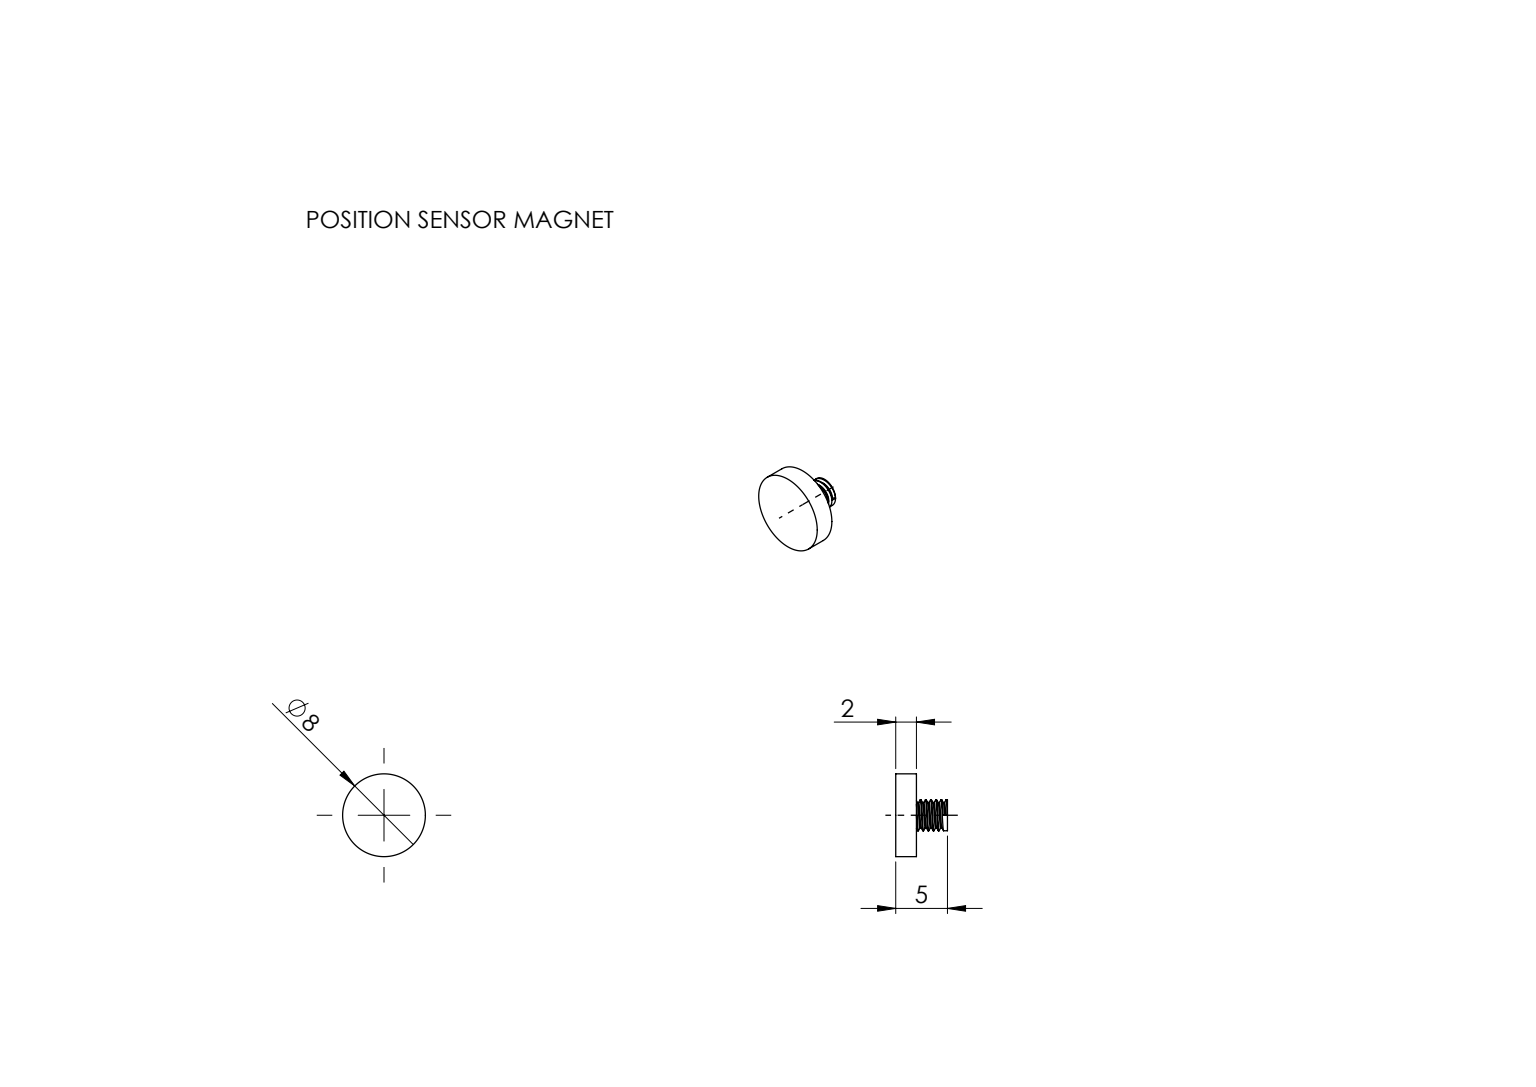
ISO-10303-21;
HEADER;
FILE_DESCRIPTION (('STEP AP214'),
    '1' );
FILE_NAME ('position sensor magnet.step',
    '2026-10-03T18:28:46',
    ( '' ),
    ( '' ),
    'SwSTEP 2.0',
    'SolidWorks 2026',
    '' );
FILE_SCHEMA (( 'AUTOMOTIVE_DESIGN' ));
ENDSEC;

DATA;
#7=EDGE_CURVE ( 'NONE', #9588, #252, #7094, .T. ) ;
#20=CARTESIAN_POINT ( 'NONE',  ( -1.500000000000000222, -13.00000000000000533, -1.812500001365593416 ) ) ;
#22=DIRECTION ( 'NONE',  ( 0.000000000000000000, 0.000000000000000000, 1.000000000000000000 ) ) ;
#32=CARTESIAN_POINT ( 'NONE',  ( -3.181725716174720498E-16, -14.73205080756888385, -1.125000000000000000 ) ) ;
#45=ORIENTED_EDGE ( 'NONE', *, *, #5401, .F. ) ;
#47=CARTESIAN_POINT ( 'NONE',  ( 1.229367062500000163, -13.00000000000000533, 0.2187499993172034862 ) ) ;
#53=CARTESIAN_POINT ( 'NONE',  ( 1.060575238724907038E-16, -11.26794919243112680, 0.06249999863440621611 ) ) ;
#66=CARTESIAN_POINT ( 'NONE',  ( 1.229367062500000385, -12.29022459553277002, -0.8020833340161301894 ) ) ;
#96=( NAMED_UNIT ( * ) PLANE_ANGLE_UNIT ( ) SI_UNIT ( $, .RADIAN. ) );
#98=ORIENTED_EDGE ( 'NONE', *, *, #3375, .T. ) ;
#106=CARTESIAN_POINT ( 'NONE',  ( 1.500000000000000222, -13.00000000000000533, -0.5625000013655934161 ) ) ;
#107=ADVANCED_FACE ( 'NONE', ( #5725 ), #127, .T. ) ;
#113=CARTESIAN_POINT ( 'NONE',  ( 1.060575238724907038E-16, -11.26794919243112680, -0.9375000013655935271 ) ) ;
#116=CARTESIAN_POINT ( 'NONE',  ( 0.6146835312500001924, -11.93533689329915326, -2.760416667349463449 ) ) ;
#127=CYLINDRICAL_SURFACE ( 'NONE', #2700, 1.500000000000000222 ) ;
#135=ORIENTED_EDGE ( 'NONE', *, *, #264, .F. ) ;
#143=CARTESIAN_POINT ( 'NONE',  ( 1.500000000000000222, -13.00000000000000533, 0.000000000000000000 ) ) ;
#148=ADVANCED_FACE ( 'NONE', ( #6475 ), #9031, .T. ) ;
#161=ADVANCED_FACE ( 'NONE', ( #10045 ), #7492, .F. ) ;
#163=CARTESIAN_POINT ( 'NONE',  ( 1.229367062500000163, -13.00000000000000533, -0.3437500006827965970 ) ) ;
#206=CYLINDRICAL_SURFACE ( 'NONE', #9839, 1.500000000000000222 ) ;
#212=CARTESIAN_POINT ( 'NONE',  ( -2.607672531582950546E-16, -14.41955080893447416, -0.3437500006827965415 ) ) ;
#215=EDGE_CURVE ( 'NONE', #8955, #6611, #5198, .T. ) ;
#217=DIRECTION ( 'NONE',  ( 1.000000000000000000, 0.000000000000000000, 0.000000000000000000 ) ) ;
#222=CARTESIAN_POINT ( 'NONE',  ( -1.229367062500000163, -13.70977540446723708, -1.052083334016129967 ) ) ;
#228=DIRECTION ( 'NONE',  ( 1.000000000000000000, 0.000000000000000000, -0.000000000000000000 ) ) ;
#252=VERTEX_POINT ( 'NONE', #2821 ) ;
#260=VECTOR ( 'NONE', #2715, 1000.000000000000000 ) ;
#263=CARTESIAN_POINT ( 'NONE',  ( -2.607672531582950546E-16, -14.41955080893447416, -1.343750000682796708 ) ) ;
#264=EDGE_CURVE ( 'NONE', #5062, #6335, #3411, .T. ) ;
#268=LINE ( 'NONE', #4231, #6080 ) ;
#272=CARTESIAN_POINT ( 'NONE',  ( -1.229367062500000163, -13.00000000000000533, -0.5937500006827968191 ) ) ;
#274=VERTEX_POINT ( 'NONE', #5981 ) ;
#276=DIRECTION ( 'NONE',  ( 1.000000000000000000, 0.000000000000000000, 0.000000000000000000 ) ) ;
#279=CARTESIAN_POINT ( 'NONE',  ( 0.9270509719278221539, -11.80318232062615991, 0.01099716686063855267 ) ) ;
#289=CARTESIAN_POINT ( 'NONE',  ( -1.229367062500000163, -13.00000000000000533, -1.468750000682796486 ) ) ;
#301=CARTESIAN_POINT ( 'NONE',  ( -1.229367062500000163, -13.00000000000000533, -2.593750000682796486 ) ) ;
#312=CARTESIAN_POINT ( 'NONE',  ( 8.692241771943169307E-17, -11.58044919106553294, -0.09375000068279677745 ) ) ;
#320=CARTESIAN_POINT ( 'NONE',  ( -2.607672531582950546E-16, -14.41955080893447416, -0.4687500006827967081 ) ) ;
#334=CARTESIAN_POINT ( 'NONE',  ( 1.229367062499999719, -13.70977540446724063, -2.260416667349463005 ) ) ;
#336=CARTESIAN_POINT ( 'NONE',  ( -2.607672531582950546E-16, -14.41955080893447416, -0.3437500006827965415 ) ) ;
#339=ORIENTED_EDGE ( 'NONE', *, *, #9880, .F. ) ;
#343=EDGE_CURVE ( 'NONE', #9521, #8355, #5353, .T. ) ;
#351=CARTESIAN_POINT ( 'NONE',  ( -0.6146835312500006365, -14.06466310670085562, -0.01041666734946352160 ) ) ;
#366=CARTESIAN_POINT ( 'NONE',  ( 1.229367062500000163, -13.00000000000000533, -2.218750000682796486 ) ) ;
#367=EDGE_LOOP ( 'NONE', ( #135, #7776, #8041, #9114 ) ) ;
#374=CARTESIAN_POINT ( 'NONE',  ( -1.229367062500000163, -12.29022459553277002, -2.635416667349463449 ) ) ;
#389=CARTESIAN_POINT ( 'NONE',  ( 1.229367062500000163, -13.00000000000000533, -1.718750000682796486 ) ) ;
#401=CARTESIAN_POINT ( 'NONE',  ( 1.229367062500000163, -13.00000000000000533, 0.1562499993172034307 ) ) ;
#415=( BOUNDED_CURVE ( )  B_SPLINE_CURVE ( 2, ( #2838, #7109, #4670, #2788, #2741, #9258, #6005 ),
 .UNSPECIFIED., .F., .T. ) 
 B_SPLINE_CURVE_WITH_KNOTS ( ( 3, 2, 2, 3 ),
 ( 0.7500000000000000000, 0.7777777777777777901, 0.8055555555555554692, 0.8333333333333332593 ),
 .UNSPECIFIED. ) 
 CURVE ( )  GEOMETRIC_REPRESENTATION_ITEM ( )  RATIONAL_B_SPLINE_CURVE ( ( 1.000000000000000000, 0.8660254037844387076, 1.000000000000000000, 0.8660254037844387076, 1.000000000000000000, 0.8660254037844392627, 0.9999999999999994449 ) ) 
 REPRESENTATION_ITEM ( '' )  );
#416=CARTESIAN_POINT ( 'NONE',  ( -1.500000000000000222, -13.00000000000000533, -1.312500001365593416 ) ) ;
#428=AXIS2_PLACEMENT_3D ( 'NONE', #1380, #3660, #8440 ) ;
#439=CARTESIAN_POINT ( 'NONE',  ( 1.229367062500000385, -12.29022459553277002, -1.677083334016129967 ) ) ;
#452=CARTESIAN_POINT ( 'NONE',  ( 0.7500000000000003331, -11.70096189432334732, -2.916666666666666963 ) ) ;
#487=CARTESIAN_POINT ( 'NONE',  ( -2.607672531582950546E-16, -14.41955080893447416, -1.968750000682796708 ) ) ;
#489=CARTESIAN_POINT ( 'NONE',  ( 8.692241771943170539E-17, -11.58044919106553650, -1.593750000682796708 ) ) ;
#499=CARTESIAN_POINT ( 'NONE',  ( -1.229367062500000385, -13.70977540446723886, -1.552083334016130189 ) ) ;
#517=CARTESIAN_POINT ( 'NONE',  ( 1.499999999999999778, -13.86602540378444637, -2.541666666666666963 ) ) ;
#531=CARTESIAN_POINT ( 'NONE',  ( 1.229367062500000163, -13.00000000000000533, -2.718750000682796486 ) ) ;
#534=CARTESIAN_POINT ( 'NONE',  ( -1.500000000000000666, -13.86602540378444637, -0.2083333333333333703 ) ) ;
#540=CARTESIAN_POINT ( 'NONE',  ( 1.229367062500000385, -12.29022459553277002, -1.802083334016129967 ) ) ;
#543=CARTESIAN_POINT ( 'NONE',  ( -1.229367062500000163, -12.29022459553277002, -1.010416667349463227 ) ) ;
#554=CARTESIAN_POINT ( 'NONE',  ( -0.6146835312500006365, -14.06466310670085562, -1.010416667349463227 ) ) ;
#560=ORIENTED_EDGE ( 'NONE', *, *, #5898, .F. ) ;
#564=CARTESIAN_POINT ( 'NONE',  ( 1.500000000000000222, -12.13397459621556784, -1.458333333333333481 ) ) ;
#581=( GEOMETRIC_REPRESENTATION_CONTEXT ( 3 ) GLOBAL_UNCERTAINTY_ASSIGNED_CONTEXT ( ( #4844 ) ) GLOBAL_UNIT_ASSIGNED_CONTEXT ( ( #7026, #8784, #10332 ) ) REPRESENTATION_CONTEXT ( 'NONE', 'WORKASPACE' ) );
#588=CARTESIAN_POINT ( 'NONE',  ( -2.607672531582950546E-16, -14.41955080893447416, -2.468750000682796486 ) ) ;
#606=CARTESIAN_POINT ( 'NONE',  ( -0.7500000000000007772, -14.29903810567666156, -1.666666666666666741 ) ) ;
#639=CARTESIAN_POINT ( 'NONE',  ( -1.229367062500000163, -13.00000000000000533, 0.03124999931720332663 ) ) ;
#647=CARTESIAN_POINT ( 'NONE',  ( 1.500000000000000222, -13.00000000000000533, 0.4374999986344065284 ) ) ;
#650=ORIENTED_EDGE ( 'NONE', *, *, #2389, .T. ) ;
#655=CARTESIAN_POINT ( 'NONE',  ( 1.500000000000000222, -13.00000000000000533, -1.500000000000000000 ) ) ;
#665=CARTESIAN_POINT ( 'NONE',  ( 0.000000000000000000, -13.00000000000000533, -3.000000000000000000 ) ) ;
#679=ORIENTED_EDGE ( 'NONE', *, *, #5695, .T. ) ;
#685=CARTESIAN_POINT ( 'NONE',  ( 0.7500000000000003331, -11.70096189432334732, 0.02083333196773980503 ) ) ;
#687=CARTESIAN_POINT ( 'NONE',  ( -1.500000000000000222, -13.00000000000000533, -0.3125000013655936937 ) ) ;
#690=ORIENTED_EDGE ( 'NONE', *, *, #6660, .T. ) ;
#700=CARTESIAN_POINT ( 'NONE',  ( 0.6146835312499993043, -14.06466310670085562, 0.1979166659838698661 ) ) ;
#708=EDGE_LOOP ( 'NONE', ( #5948, #2687, #4855, #10434, #9641, #7515, #7392, #3265, #7780, #4226, #690, #4016, #8469, #9796, #6235 ) ) ;
#716=CARTESIAN_POINT ( 'NONE',  ( 0.7500000000000003331, -11.70096189432334732, -0.9166666666666667407 ) ) ;
#740=CARTESIAN_POINT ( 'NONE',  ( -0.7499999999999997780, -11.70096189432334555, -0.3958333346989269530 ) ) ;
#741=CIRCLE ( 'NONE', #9725, 4.000000000000000000 ) ;
#748=EDGE_CURVE ( 'NONE', #10270, #6751, #4270, .T. ) ;
#758=DIRECTION ( 'NONE',  ( 0.000000000000000000, 0.000000000000000000, 1.000000000000000000 ) ) ;
#764=DIRECTION ( 'NONE',  ( 1.000000000000000000, 0.000000000000000000, 0.000000000000000000 ) ) ;
#768=CARTESIAN_POINT ( 'NONE',  ( 1.060575238724907038E-16, -11.26794919243112680, -0.8750000000000004441 ) ) ;
#774=CIRCLE ( 'NONE', #8227, 1.500000000000000222 ) ;
#775=CARTESIAN_POINT ( 'NONE',  ( 1.500000000000000222, -12.13397459621556784, -2.520833334698926897 ) ) ;
#788=CARTESIAN_POINT ( 'NONE',  ( -1.499999999999998224, -12.13397459621556607, -1.791666666666667185 ) ) ;
#794=CARTESIAN_POINT ( 'NONE',  ( 1.500000000000000444, -12.13397459621556607, -0.5208333346989270085 ) ) ;
#797=ADVANCED_FACE ( 'NONE', ( #10440 ), #5240, .T. ) ;
#806=CARTESIAN_POINT ( 'NONE',  ( -0.6146835312499998594, -11.93533689329915326, -0.6770833340161300784 ) ) ;
#815=CARTESIAN_POINT ( 'NONE',  ( 0.000000000000000000, -13.00000000000000533, 0.000000000000000000 ) ) ;
#819=CARTESIAN_POINT ( 'NONE',  ( -1.500000000000000000, -12.13397459621556607, -1.791666666666666741 ) ) ;
#820=ORIENTED_EDGE ( 'NONE', *, *, #940, .F. ) ;
#828=EDGE_CURVE ( 'NONE', #5863, #2098, #3844, .T. ) ;
#829=VECTOR ( 'NONE', #7182, 1000.000000000000227 ) ;
#844=CARTESIAN_POINT ( 'NONE',  ( -1.500000000000000666, -13.86602540378444459, -0.2708333346989268420 ) ) ;
#849=CARTESIAN_POINT ( 'NONE',  ( -1.500000000000000222, -13.00000000000000533, -0.8125000013655935271 ) ) ;
#859=EDGE_CURVE ( 'NONE', #6218, #8785, #9534, .T. ) ;
#860=CARTESIAN_POINT ( 'NONE',  ( -2.607672531582950546E-16, -14.41955080893447416, -0.9687500006827967081 ) ) ;
#871=AXIS2_PLACEMENT_3D ( 'NONE', #3735, #4797, #7928 ) ;
#879=CARTESIAN_POINT ( 'NONE',  ( -0.6146835312499998594, -11.93533689329915326, -2.552083334016129967 ) ) ;
#884=ORIENTED_EDGE ( 'NONE', *, *, #6432, .T. ) ;
#885=EDGE_CURVE ( 'NONE', #4827, #274, #3898, .T. ) ;
#898=CARTESIAN_POINT ( 'NONE',  ( -1.500000000000000222, -13.00000000000000533, -1.312500001365593416 ) ) ;
#904=FACE_OUTER_BOUND ( 'NONE', #4621, .T. ) ;
#907=CARTESIAN_POINT ( 'NONE',  ( 1.229367062500000163, -12.29022459553277002, -2.802083334016129967 ) ) ;
#910=CARTESIAN_POINT ( 'NONE',  ( -1.229367062500000163, -12.29022459553277002, -1.135416667349463227 ) ) ;
#927=( GEOMETRIC_REPRESENTATION_CONTEXT ( 3 ) GLOBAL_UNCERTAINTY_ASSIGNED_CONTEXT ( ( #6427 ) ) GLOBAL_UNIT_ASSIGNED_CONTEXT ( ( #1683, #96, #6600 ) ) REPRESENTATION_CONTEXT ( 'NONE', 'WORKASPACE' ) );
#938=CARTESIAN_POINT ( 'NONE',  ( 1.499999999999999778, -13.86602540378444637, -1.104166668032260379 ) ) ;
#940=EDGE_CURVE ( 'NONE', #2098, #9635, #9900, .T. ) ;
#958=ORIENTED_EDGE ( 'NONE', *, *, #5876, .F. ) ;
#960=CARTESIAN_POINT ( 'NONE',  ( 0.6146835312499993043, -14.06466310670085562, -1.427083334016129967 ) ) ;
#987=CARTESIAN_POINT ( 'NONE',  ( 1.500000000000000222, -13.00000000000000533, -1.062500001365593416 ) ) ;
#988=ORIENTED_EDGE ( 'NONE', *, *, #5006, .F. ) ;
#989=ORIENTED_EDGE ( 'NONE', *, *, #6351, .F. ) ;
#997=CARTESIAN_POINT ( 'NONE',  ( -0.6146835312499998594, -11.93533689329915326, -0.5520833340161299674 ) ) ;
#1006=CARTESIAN_POINT ( 'NONE',  ( 1.229367062500000163, -13.00000000000000533, -0.8437500006827965970 ) ) ;
#1017=FACE_OUTER_BOUND ( 'NONE', #1736, .T. ) ;
#1020=CARTESIAN_POINT ( 'NONE',  ( -1.229367062500000163, -12.29022459553277002, -1.510416667349463227 ) ) ;
#1030=AXIS2_PLACEMENT_3D ( 'NONE', #8223, #1546, #7416 ) ;
#1033=EDGE_CURVE ( 'NONE', #1639, #6225, #3260, .T. ) ;
#1042=CARTESIAN_POINT ( 'NONE',  ( 1.229367062500000163, -13.00000000000000533, -2.343750000682796486 ) ) ;
#1054=CARTESIAN_POINT ( 'NONE',  ( -1.229367062500000163, -13.00000000000000533, -1.468750000682796486 ) ) ;
#1061=VERTEX_POINT ( 'NONE', #6314 ) ;
#1063=CARTESIAN_POINT ( 'NONE',  ( -1.229367062500000163, -12.29022459553277002, -0.6354166673494632267 ) ) ;
#1074=CARTESIAN_POINT ( 'NONE',  ( 1.500000000000000222, -13.00000000000000533, -3.000000000000000000 ) ) ;
#1076=CARTESIAN_POINT ( 'NONE',  ( 0.6146835312500001924, -11.93533689329915326, -2.135416667349463449 ) ) ;
#1079=CARTESIAN_POINT ( 'NONE',  ( 1.229367062500000163, -13.00000000000000533, -2.218750000682796486 ) ) ;
#1089=CARTESIAN_POINT ( 'NONE',  ( 1.229367062500000385, -12.29022459553277002, -2.802083334016129523 ) ) ;
#1095=CARTESIAN_POINT ( 'NONE',  ( -1.500000000000000222, -13.00000000000000533, -0.2500000000000002220 ) ) ;
#1101=CARTESIAN_POINT ( 'NONE',  ( 8.692241771943169307E-17, -11.58044919106553294, -1.593750000682796486 ) ) ;
#1106=CARTESIAN_POINT ( 'NONE',  ( -1.500000000000000222, -13.00000000000000533, -2.750000000000000000 ) ) ;
#1107=CARTESIAN_POINT ( 'NONE',  ( -1.499999999999996669, -12.13397459621556607, -0.8541666680322607119 ) ) ;
#1112=CARTESIAN_POINT ( 'NONE',  ( -1.229367062500000163, -13.00000000000000533, -2.093750000682796930 ) ) ;
#1128=CARTESIAN_POINT ( 'NONE',  ( 0.6146835312500001924, -11.93533689329915326, -1.135416667349463227 ) ) ;
#1131=CARTESIAN_POINT ( 'NONE',  ( 0.6146835312499993043, -14.06466310670085562, -1.802083334016129745 ) ) ;
#1151=CARTESIAN_POINT ( 'NONE',  ( -2.607672531582950546E-16, -14.41955080893447416, 0.1562499993172034585 ) ) ;
#1152=EDGE_CURVE ( 'NONE', #4358, #7070, #4378, .T. ) ;
#1160=CARTESIAN_POINT ( 'NONE',  ( -1.229367062500000163, -13.00000000000000533, -1.593750000682796708 ) ) ;
#1176=CARTESIAN_POINT ( 'NONE',  ( -0.6146835312500006365, -14.06466310670085562, -0.8854166673494632267 ) ) ;
#1178=CARTESIAN_POINT ( 'NONE',  ( -1.229367062500000163, -13.00000000000000533, -0.4687500006827967081 ) ) ;
#1181=COLOUR_RGB ( '', 0.09019608, 0.27058824, 0.51372549) ;
#1192=CARTESIAN_POINT ( 'NONE',  ( 0.6146835312499993043, -14.06466310670085562, 0.07291666598386974119 ) ) ;
#1195=VECTOR ( 'NONE', #7864, 1000.000000000000000 ) ;
#1202=ORIENTED_EDGE ( 'NONE', *, *, #1450, .T. ) ;
#1229=CARTESIAN_POINT ( 'NONE',  ( -0.6146835312499998594, -11.93533689329915326, -2.052083334016129967 ) ) ;
#1231=CARTESIAN_POINT ( 'NONE',  ( -0.6146835312499998594, -11.93533689329915326, -2.052083334016129967 ) ) ;
#1246=CARTESIAN_POINT ( 'NONE',  ( -0.6146835312499998594, -11.93533689329915326, -0.1770833340161300506 ) ) ;
#1261=ORIENTED_EDGE ( 'NONE', *, *, #9693, .T. ) ;
#1264=DIRECTION ( 'NONE',  ( 1.000000000000000000, 0.000000000000000000, 0.000000000000000000 ) ) ;
#1276=PRODUCT_DEFINITION ( 'UNKNOWN', '', #9579, #7173 ) ;
#1282=CARTESIAN_POINT ( 'NONE',  ( -1.229367062500000163, -12.29022459553277002, -0.01041666734946308792 ) ) ;
#1284=CARTESIAN_POINT ( 'NONE',  ( 1.229367062500000163, -13.00000000000000533, -0.2187500006827964583 ) ) ;
#1294=PRESENTATION_STYLE_ASSIGNMENT (( #8606 ) ) ;
#1296=CARTESIAN_POINT ( 'NONE',  ( -0.6146835312500006365, -14.06466310670085562, -2.010416667349463005 ) ) ;
#1312=DIRECTION ( 'NONE',  ( 0.000000000000000000, 0.000000000000000000, 1.000000000000000000 ) ) ;
#1328=CARTESIAN_POINT ( 'NONE',  ( -0.6146835312500006365, -14.06466310670085562, 0.1145833326505365929 ) ) ;
#1330=CARTESIAN_POINT ( 'NONE',  ( -1.229367062500000163, -13.70977540446723708, -1.427083334016129745 ) ) ;
#1341=ADVANCED_FACE ( 'NONE', ( #6840 ), #10110, .T. ) ;
#1346=CARTESIAN_POINT ( 'NONE',  ( 1.229367062500000385, -12.29022459553277002, -1.302083334016129967 ) ) ;
#1365=DIRECTION ( 'NONE',  ( 0.000000000000000000, 0.000000000000000000, 1.000000000000000000 ) ) ;
#1366=AXIS2_PLACEMENT_3D ( 'NONE', #3051, #8669, #1515 ) ;
#1372=VERTEX_POINT ( 'NONE', #8916 ) ;
#1380=CARTESIAN_POINT ( 'NONE',  ( 0.000000000000000000, -13.00000000000000533, -3.000000000000000000 ) ) ;
#1386=CARTESIAN_POINT ( 'NONE',  ( 0.6146835312499993043, -14.06466310670085562, -1.927083334016129967 ) ) ;
#1400=CARTESIAN_POINT ( 'NONE',  ( 1.500000000000000000, -13.86602540378444459, -0.04166666666666684476 ) ) ;
#1424=CARTESIAN_POINT ( 'NONE',  ( 1.060575238724907038E-16, -11.26794919243112680, -1.937500001365593416 ) ) ;
#1427=( BOUNDED_CURVE ( )  B_SPLINE_CURVE ( 2, ( #7646, #9285, #7539, #8545, #9987, #1871, #8394 ),
 .UNSPECIFIED., .F., .T. ) 
 B_SPLINE_CURVE_WITH_KNOTS ( ( 3, 2, 2, 3 ),
 ( 0.1666666666666666574, 0.1944444444444444475, 0.2222222222222222099, 0.2500000000000000000 ),
 .UNSPECIFIED. ) 
 CURVE ( )  GEOMETRIC_REPRESENTATION_ITEM ( )  RATIONAL_B_SPLINE_CURVE ( ( 1.000000000000000000, 0.8660254037844387076, 1.000000000000000000, 0.8660254037844387076, 1.000000000000000000, 0.8660254037844387076, 1.000000000000000000 ) ) 
 REPRESENTATION_ITEM ( '' )  );
#1433=VECTOR ( 'NONE', #6619, 1000.000000000000000 ) ;
#1438=CARTESIAN_POINT ( 'NONE',  ( 1.229367062500000385, -12.29022459553277002, -0.6770833340161300784 ) ) ;
#1450=EDGE_CURVE ( 'NONE', #7070, #4358, #9157, .T. ) ;
#1453=AXIS2_PLACEMENT_3D ( 'NONE', #4245, #22, #5722 ) ;
#1456=CARTESIAN_POINT ( 'NONE',  ( -0.7499999999999997780, -11.70096189432334555, -0.8333333333333334814 ) ) ;
#1465=CARTESIAN_POINT ( 'NONE',  ( -2.607672531582950546E-16, -14.41955080893447416, 0.03124999931720332663 ) ) ;
#1479=CARTESIAN_POINT ( 'NONE',  ( -1.229367062500000385, -13.70977540446723886, -2.427083334016129967 ) ) ;
#1487=CARTESIAN_POINT ( 'NONE',  ( -1.500000000000000222, -13.00000000000000533, -2.250000000000000444 ) ) ;
#1492=CARTESIAN_POINT ( 'NONE',  ( 1.229367062500000385, -12.29022459553277002, -1.302083334016129967 ) ) ;
#1493=( BOUNDED_CURVE ( )  B_SPLINE_CURVE ( 2, ( #6137, #3861, #7089, #7949, #9387, #2918, #687 ),
 .UNSPECIFIED., .F., .T. ) 
 B_SPLINE_CURVE_WITH_KNOTS ( ( 3, 2, 2, 3 ),
 ( 0.6666666666666666297, 0.6944444444444444198, 0.7222222222222222099, 0.7500000000000000000 ),
 .UNSPECIFIED. ) 
 CURVE ( )  GEOMETRIC_REPRESENTATION_ITEM ( )  RATIONAL_B_SPLINE_CURVE ( ( 1.000000000000000000, 0.8660254037844387076, 1.000000000000000000, 0.8660254037844387076, 1.000000000000000000, 0.8660254037844387076, 1.000000000000000000 ) ) 
 REPRESENTATION_ITEM ( '' )  );
#1506=CARTESIAN_POINT ( 'NONE',  ( -0.7500000000000007772, -14.29903810567666156, -0.2291666680322604066 ) ) ;
#1509=CARTESIAN_POINT ( 'NONE',  ( 0.7500000000000003331, -11.70096189432334732, -1.916666666666666741 ) ) ;
#1510=AXIS2_PLACEMENT_3D ( 'NONE', #665, #1520, #3953 ) ;
#1511=EDGE_LOOP ( 'NONE', ( #7554, #6393 ) ) ;
#1514=( BOUNDED_CURVE ( )  B_SPLINE_CURVE ( 2, ( #2301, #5470, #7818, #3831, #9572, #2352, #10308 ),
 .UNSPECIFIED., .F., .T. ) 
 B_SPLINE_CURVE_WITH_KNOTS ( ( 3, 2, 2, 3 ),
 ( 0.4166666666666666297, 0.4444444444444443643, 0.4722222222222222099, 0.5000000000000000000 ),
 .UNSPECIFIED. ) 
 CURVE ( )  GEOMETRIC_REPRESENTATION_ITEM ( )  RATIONAL_B_SPLINE_CURVE ( ( 1.000000000000000222, 0.8660254037844384856, 1.000000000000000000, 0.8660254037844387076, 1.000000000000000000, 0.8660254037844387076, 1.000000000000000000 ) ) 
 REPRESENTATION_ITEM ( '' )  );
#1515=DIRECTION ( 'NONE',  ( 1.000000000000000000, 0.000000000000000000, 0.000000000000000000 ) ) ;
#1520=DIRECTION ( 'NONE',  ( 0.000000000000000000, 0.000000000000000000, 1.000000000000000000 ) ) ;
#1532=EDGE_LOOP ( 'NONE', ( #6973, #5382, #7121, #4739 ) ) ;
#1538=CARTESIAN_POINT ( 'NONE',  ( 1.500000000000000000, -13.86602540378444459, 0.3958333319677397322 ) ) ;
#1543=CIRCLE ( 'NONE', #871, 1.500000000000000222 ) ;
#1544=CARTESIAN_POINT ( 'NONE',  ( 1.499999999999999778, -13.86602540378444637, -0.6041666680322602678 ) ) ;
#1546=DIRECTION ( 'NONE',  ( 0.000000000000000000, 0.000000000000000000, 1.000000000000000000 ) ) ;
#1560=CARTESIAN_POINT ( 'NONE',  ( 0.000000000000000000, -13.00000000000000533, 2.000000000000000000 ) ) ;
#1561=ORIENTED_EDGE ( 'NONE', *, *, #6420, .F. ) ;
#1570=CARTESIAN_POINT ( 'NONE',  ( 1.060575238724907038E-16, -11.26794919243112680, -1.375000000000000222 ) ) ;
#1576=CARTESIAN_POINT ( 'NONE',  ( -1.500000000000000222, -13.00000000000000533, -3.000000000000000000 ) ) ;
#1578=ORIENTED_EDGE ( 'NONE', *, *, #9879, .T. ) ;
#1587=DIRECTION ( 'NONE',  ( -0.000000000000000000, -0.000000000000000000, 1.000000000000000000 ) ) ;
#1594=CARTESIAN_POINT ( 'NONE',  ( 0.7499999999999991118, -14.29903810567666333, -0.1458333346989267310 ) ) ;
#1600=CARTESIAN_POINT ( 'NONE',  ( 1.499999999999999778, -13.86602540378444637, -2.041666666666666963 ) ) ;
#1605=CARTESIAN_POINT ( 'NONE',  ( -1.229367062500000163, -13.00000000000000533, -0.09375000068279679133 ) ) ;
#1619=CARTESIAN_POINT ( 'NONE',  ( 1.500000000000000222, -13.00000000000000533, -1.000000000000000000 ) ) ;
#1639=VERTEX_POINT ( 'NONE', #6985 ) ;
#1644=CARTESIAN_POINT ( 'NONE',  ( -0.7499999999999997780, -11.70096189432334555, -1.395833334698926897 ) ) ;
#1668=CARTESIAN_POINT ( 'NONE',  ( -1.229367062500000163, -13.00000000000000533, -2.468750000682796486 ) ) ;
#1683=( LENGTH_UNIT ( ) NAMED_UNIT ( * ) SI_UNIT ( .MILLI., .METRE. ) );
#1695=CARTESIAN_POINT ( 'NONE',  ( -0.7500000000000007772, -14.29903810567666156, 0.2708333319677396211 ) ) ;
#1698=DIRECTION ( 'NONE',  ( 0.000000000000000000, 0.000000000000000000, 1.000000000000000000 ) ) ;
#1699=FACE_OUTER_BOUND ( 'NONE', #7725, .T. ) ;
#1716=CARTESIAN_POINT ( 'NONE',  ( 1.500000000000000222, -13.00000000000000533, -1.562500001365593416 ) ) ;
#1735=CARTESIAN_POINT ( 'NONE',  ( -1.229367062500000385, -13.70977540446723886, -2.552083334016129967 ) ) ;
#1736=EDGE_LOOP ( 'NONE', ( #10338, #679, #7987, #4069 ) ) ;
#1745=CARTESIAN_POINT ( 'NONE',  ( 1.229367062500000385, -12.29022459553277002, -0.1770833340161300229 ) ) ;
#1750=CARTESIAN_POINT ( 'NONE',  ( 1.500000000000000222, -13.00000000000000533, -1.062500001365593416 ) ) ;
#1752=DIRECTION ( 'NONE',  ( 0.000000000000000000, 0.000000000000000000, 1.000000000000000000 ) ) ;
#1755=CARTESIAN_POINT ( 'NONE',  ( -0.6146835312500006365, -14.06466310670085562, -2.510416667349463005 ) ) ;
#1765=ADVANCED_FACE ( 'NONE', ( #10189 ), #7590, .T. ) ;
#1773=ORIENTED_EDGE ( 'NONE', *, *, #7796, .T. ) ;
#1774=( BOUNDED_CURVE ( )  B_SPLINE_CURVE ( 2, ( #10278, #3847, #7732, #2955, #3007, #7883, #416 ),
 .UNSPECIFIED., .F., .T. ) 
 B_SPLINE_CURVE_WITH_KNOTS ( ( 3, 2, 2, 3 ),
 ( 0.3333333333333333148, 0.3611111111111111049, 0.3888888888888888395, 0.4166666666666666297 ),
 .UNSPECIFIED. ) 
 CURVE ( )  GEOMETRIC_REPRESENTATION_ITEM ( )  RATIONAL_B_SPLINE_CURVE ( ( 1.000000000000000000, 0.8660254037844387076, 1.000000000000000000, 0.8660254037844387076, 1.000000000000000000, 0.8660254037844389297, 0.9999999999999997780 ) ) 
 REPRESENTATION_ITEM ( '' )  );
#1800=CARTESIAN_POINT ( 'NONE',  ( 1.229367062500000163, -13.00000000000000533, -1.718750000682796486 ) ) ;
#1805=CARTESIAN_POINT ( 'NONE',  ( -1.500000000000000222, -13.00000000000000533, -0.8125000013655935271 ) ) ;
#1806=ORIENTED_EDGE ( 'NONE', *, *, #3812, .F. ) ;
#1808=CARTESIAN_POINT ( 'NONE',  ( -1.229367062500000163, -12.29022459553277002, -1.135416667349463449 ) ) ;
#1822=CARTESIAN_POINT ( 'NONE',  ( -1.229367062500000163, -12.29022459553277002, -2.010416667349463005 ) ) ;
#1824=CARTESIAN_POINT ( 'NONE',  ( 8.692241771943170539E-17, -11.58044919106553650, -2.593750000682796486 ) ) ;
#1835=EDGE_CURVE ( 'NONE', #6218, #9020, #1774, .T. ) ;
#1836=( BOUNDED_CURVE ( )  B_SPLINE_CURVE ( 2, ( #4860, #6497, #10451, #5603, #8105, #788, #4018 ),
 .UNSPECIFIED., .F., .T. ) 
 B_SPLINE_CURVE_WITH_KNOTS ( ( 3, 2, 2, 3 ),
 ( 0.3333333333333333148, 0.3611111111111111049, 0.3888888888888888395, 0.4166666666666666297 ),
 .UNSPECIFIED. ) 
 CURVE ( )  GEOMETRIC_REPRESENTATION_ITEM ( )  RATIONAL_B_SPLINE_CURVE ( ( 1.000000000000000000, 0.8660254037844387076, 1.000000000000000000, 0.8660254037844387076, 1.000000000000000000, 0.8660254037844389297, 0.9999999999999997780 ) ) 
 REPRESENTATION_ITEM ( '' )  );
#1837=CARTESIAN_POINT ( 'NONE',  ( -1.229367062500000163, -12.29022459553277002, -2.635416667349463449 ) ) ;
#1849=CARTESIAN_POINT ( 'NONE',  ( -1.229367062500000163, -12.29022459553277002, -0.01041666734946308792 ) ) ;
#1860=CARTESIAN_POINT ( 'NONE',  ( -1.229367062500000163, -13.70977540446723708, -2.552083334016129967 ) ) ;
#1871=CARTESIAN_POINT ( 'NONE',  ( -1.499999999999999778, -12.13397459621556784, -1.854166668032260379 ) ) ;
#1874=CARTESIAN_POINT ( 'NONE',  ( -2.607672531582950546E-16, -14.41955080893447416, -1.843750000682796708 ) ) ;
#1879=ORIENTED_EDGE ( 'NONE', *, *, #264, .T. ) ;
#1899=EDGE_CURVE ( 'NONE', #8785, #9003, #3936, .T. ) ;
#1905=CARTESIAN_POINT ( 'NONE',  ( 1.229367062500000163, -13.00000000000000533, -0.7187500006827964860 ) ) ;
#1914=CARTESIAN_POINT ( 'NONE',  ( 1.229367062500000163, -13.00000000000000533, -2.343750000682796486 ) ) ;
#1930=CARTESIAN_POINT ( 'NONE',  ( -1.229367062500000163, -12.29022459553277002, -0.5104166673494631157 ) ) ;
#1931=ORIENTED_EDGE ( 'NONE', *, *, #7531, .T. ) ;
#1954=CARTESIAN_POINT ( 'NONE',  ( -1.229367062500000163, -13.00000000000000533, -0.9687500006827964860 ) ) ;
#1965=CARTESIAN_POINT ( 'NONE',  ( -1.229367062500000163, -13.00000000000000533, -0.09375000068279679133 ) ) ;
#1972=CARTESIAN_POINT ( 'NONE',  ( -0.7499999999999997780, -11.70096189432334555, 0.1041666653010730748 ) ) ;
#1974=CARTESIAN_POINT ( 'NONE',  ( 1.500000000000000222, -13.00000000000000533, 0.000000000000000000 ) ) ;
#1980=CARTESIAN_POINT ( 'NONE',  ( -1.229367062500000163, -12.29022459553277002, -1.010416667349463449 ) ) ;
#1983=CARTESIAN_POINT ( 'NONE',  ( -2.607672531582950546E-16, -14.41955080893447416, -1.343750000682796486 ) ) ;
#1993=CARTESIAN_POINT ( 'NONE',  ( -1.229367062500000385, -13.70977540446723886, -2.052083334016129967 ) ) ;
#2006=CARTESIAN_POINT ( 'NONE',  ( -0.7499999999999997780, -11.70096189432334555, -1.333333333333333481 ) ) ;
#2009=CARTESIAN_POINT ( 'NONE',  ( 1.500000000000000222, -13.00000000000000533, -2.500000000000000000 ) ) ;
#2030=CARTESIAN_POINT ( 'NONE',  ( -1.229367062500000385, -13.70977540446723886, -1.927083334016129745 ) ) ;
#2032=CARTESIAN_POINT ( 'NONE',  ( -1.229367062500000163, -13.00000000000000533, -0.9687500006827964860 ) ) ;
#2045=CARTESIAN_POINT ( 'NONE',  ( 8.692241771943169307E-17, -11.58044919106553294, -0.2187500006827968746 ) ) ;
#2065=CYLINDRICAL_SURFACE ( 'NONE', #7098, 1.500000000000000222 ) ;
#2072=CARTESIAN_POINT ( 'NONE',  ( 0.7499999999999991118, -14.29903810567666333, -2.145833334698926897 ) ) ;
#2074=CARTESIAN_POINT ( 'NONE',  ( 1.499999999999999778, -13.86602540378444637, 0.3958333319677397322 ) ) ;
#2081=CARTESIAN_POINT ( 'NONE',  ( -1.229367062500000163, -12.29022459553277002, -0.5104166673494631157 ) ) ;
#2083=CARTESIAN_POINT ( 'NONE',  ( -1.229367062500000163, -13.00000000000000533, 0.03124999931720332663 ) ) ;
#2091=CARTESIAN_POINT ( 'NONE',  ( 1.500000000000000222, -13.00000000000000533, -3.000000000000000000 ) ) ;
#2097=CARTESIAN_POINT ( 'NONE',  ( -0.7500000000000007772, -14.29903810567666156, -2.666666666666666519 ) ) ;
#2098=VERTEX_POINT ( 'NONE', #647 ) ;
#2101=AXIS2_PLACEMENT_3D ( 'NONE', #7090, #5610, #4547 ) ;
#2127=CARTESIAN_POINT ( 'NONE',  ( 1.500000000000000222, -12.13397459621556784, -2.458333333333333037 ) ) ;
#2132=CARTESIAN_POINT ( 'NONE',  ( -1.500000000000000222, -13.00000000000000533, -3.000000000000000000 ) ) ;
#2134=CARTESIAN_POINT ( 'NONE',  ( -1.229367062500000385, -13.70977540446723886, -1.552083334016130189 ) ) ;
#2138=CARTESIAN_POINT ( 'NONE',  ( 1.229367062500000163, -12.29022459553277002, -0.1770833340161300506 ) ) ;
#2150=CARTESIAN_POINT ( 'NONE',  ( 1.229367062499999719, -13.70977540446724063, -0.3854166673494633932 ) ) ;
#2155=ORIENTED_EDGE ( 'NONE', *, *, #9628, .T. ) ;
#2168=CARTESIAN_POINT ( 'NONE',  ( -1.500000000000000222, -13.00000000000000533, -1.250000000000000000 ) ) ;
#2172=CARTESIAN_POINT ( 'NONE',  ( 1.060575238724907038E-16, -11.26794919243112680, -2.437500001365593860 ) ) ;
#2173=CARTESIAN_POINT ( 'NONE',  ( 4.000000000000000000, -13.00000000000000533, 2.000000000000000000 ) ) ;
#2174=( BOUNDED_SURFACE ( )  B_SPLINE_SURFACE ( 1, 2, ( 
 ( #8997, #1089, #4312, #2632, #9101, #1837, #301, #1735, #2737, #3523, #5061, #8310, #1042, #10458, #7508, #6700, #10007, #5947, #9202, #1993, #1296, #4522, #5321, #2944, #8609, #7766, #4574, #6213, #10060, #3578, #5273, #499, #3730, #2200, #5425, #7823, #6049, #1346, #2834, #6855, #10161, #7717, #8565, #7661, #554, #2784, #6962, #8666, #3782, #5999, #9304, #6906, #7011, #6804, #10215, #6162, #4363, #9418, #5212, #2150, #8460, #9255, #8512, #2045, #1246, #10266, #7606, #5370, #351, #4418, #1192, #10111, #401 ),
 ( #3626, #4471, #452, #3679, #9467, #2887, #6111, #9362, #2097, #2997, #6267, #3945, #3048, #8087, #10430, #9578, #3153, #2308, #9632, #10313, #2358, #5476, #6379, #3099, #9738, #8828, #1509, #3836, #10376, #819, #9526, #2252, #606, #7174, #5580, #7120, #655, #3889, #8038, #1570, #8879, #6481, #3203, #8715, #9690, #32, #4794, #6319, #1619, #5531, #716, #768, #1456, #4049, #8770, #4004, #7284, #4734, #3257, #7232, #4680, #7924, #7984, #2469, #10488, #7064, #6429, #2417, #5634, #4845, #5683, #1400, #4625 ) ),
 .UNSPECIFIED., .F., .F., .T. ) 
 B_SPLINE_SURFACE_WITH_KNOTS ( ( 2, 2 ),
 ( 3, 2, 2, 2, 2, 2, 2, 2, 2, 2, 2, 2, 2, 2, 2, 2, 2, 2, 2, 2, 2, 2, 2, 2, 2, 2, 2, 2, 2, 2, 2, 2, 2, 2, 2, 2, 3 ),
 ( 0.000000000000000000, 1.000000000000000000 ),
 ( 0.000000000000000000, 0.02777777777777777624, 0.05555555555555555247, 0.08333333333333332871, 0.1111111111111111049, 0.1388888888888888951, 0.1666666666666666574, 0.1944444444444444475, 0.2222222222222222099, 0.2500000000000000000, 0.2777777777777777901, 0.3055555555555555802, 0.3333333333333333148, 0.3611111111111111049, 0.3888888888888888951, 0.4166666666666666852, 0.4444444444444444198, 0.4722222222222222099, 0.5000000000000000000, 0.5277777777777777901, 0.5555555555555555802, 0.5833333333333333703, 0.6111111111111111605, 0.6388888888888888395, 0.6666666666666666297, 0.6944444444444444198, 0.7222222222222222099, 0.7500000000000000000, 0.7777777777777777901, 0.8055555555555555802, 0.8333333333333333703, 0.8611111111111111605, 0.8888888888888888395, 0.9166666666666666297, 0.9444444444444444198, 0.9722222222222222099, 1.000000000000000000 ),
 .UNSPECIFIED. ) 
 GEOMETRIC_REPRESENTATION_ITEM ( )  RATIONAL_B_SPLINE_SURFACE ( (
 ( 1.000000000000000000, 0.8660254037844387076, 1.000000000000000000, 0.8660254037844387076, 1.000000000000000000, 0.8660254037844387076, 1.000000000000000000, 0.8660254037844387076, 1.000000000000000000, 0.8660254037844387076, 1.000000000000000000, 0.8660254037844387076, 1.000000000000000000, 0.8660254037844387076, 1.000000000000000000, 0.8660254037844387076, 1.000000000000000000, 0.8660254037844387076, 1.000000000000000000, 0.8660254037844387076, 1.000000000000000000, 0.8660254037844387076, 1.000000000000000000, 0.8660254037844387076, 1.000000000000000000, 0.8660254037844387076, 1.000000000000000000, 0.8660254037844387076, 1.000000000000000000, 0.8660254037844387076, 1.000000000000000000, 0.8660254037844387076, 1.000000000000000000, 0.8660254037844387076, 1.000000000000000000, 0.8660254037844387076, 1.000000000000000000, 0.8660254037844387076, 1.000000000000000000, 0.8660254037844387076, 1.000000000000000000, 0.8660254037844387076, 1.000000000000000000, 0.8660254037844387076, 1.000000000000000000, 0.8660254037844387076, 1.000000000000000000, 0.8660254037844387076, 1.000000000000000000, 0.8660254037844387076, 1.000000000000000000, 0.8660254037844387076, 1.000000000000000000, 0.8660254037844387076, 1.000000000000000000, 0.8660254037844387076, 1.000000000000000000, 0.8660254037844387076, 1.000000000000000000, 0.8660254037844387076, 1.000000000000000000, 0.8660254037844387076, 1.000000000000000000, 0.8660254037844387076, 1.000000000000000000, 0.8660254037844387076, 1.000000000000000000, 0.8660254037844387076, 1.000000000000000000, 0.8660254037844387076, 1.000000000000000000, 0.8660254037844387076, 1.000000000000000000),
 ( 1.000000000000000000, 0.8660254037844387076, 1.000000000000000000, 0.8660254037844387076, 1.000000000000000000, 0.8660254037844387076, 1.000000000000000000, 0.8660254037844387076, 1.000000000000000000, 0.8660254037844387076, 1.000000000000000000, 0.8660254037844387076, 1.000000000000000000, 0.8660254037844387076, 1.000000000000000000, 0.8660254037844387076, 1.000000000000000000, 0.8660254037844387076, 1.000000000000000000, 0.8660254037844387076, 1.000000000000000000, 0.8660254037844387076, 1.000000000000000000, 0.8660254037844387076, 1.000000000000000000, 0.8660254037844387076, 1.000000000000000000, 0.8660254037844387076, 1.000000000000000000, 0.8660254037844387076, 1.000000000000000000, 0.8660254037844387076, 1.000000000000000000, 0.8660254037844387076, 1.000000000000000000, 0.8660254037844387076, 1.000000000000000000, 0.8660254037844387076, 1.000000000000000000, 0.8660254037844387076, 1.000000000000000000, 0.8660254037844387076, 1.000000000000000000, 0.8660254037844387076, 1.000000000000000000, 0.8660254037844387076, 1.000000000000000000, 0.8660254037844387076, 1.000000000000000000, 0.8660254037844387076, 1.000000000000000000, 0.8660254037844387076, 1.000000000000000000, 0.8660254037844387076, 1.000000000000000000, 0.8660254037844387076, 1.000000000000000000, 0.8660254037844387076, 1.000000000000000000, 0.8660254037844387076, 1.000000000000000000, 0.8660254037844387076, 1.000000000000000000, 0.8660254037844387076, 1.000000000000000000, 0.8660254037844387076, 1.000000000000000000, 0.8660254037844387076, 1.000000000000000000, 0.8660254037844387076, 1.000000000000000000, 0.8660254037844387076, 1.000000000000000000) ) ) 
 REPRESENTATION_ITEM ( '' )  SURFACE ( )  );
#2175=LINE ( 'NONE', #7204, #5810 ) ;
#2177=CARTESIAN_POINT ( 'NONE',  ( 0.7500000000000003331, -11.70096189432334732, -2.416666666666666963 ) ) ;
#2179=CARTESIAN_POINT ( 'NONE',  ( -1.500000000000000222, -13.00000000000000533, -1.250000000000000000 ) ) ;
#2183=CARTESIAN_POINT ( 'NONE',  ( 8.692241771943169307E-17, -11.58044919106553294, -0.5937500006827968191 ) ) ;
#2189=AXIS2_PLACEMENT_3D ( 'NONE', #815, #5629, #764 ) ;
#2200=CARTESIAN_POINT ( 'NONE',  ( -2.607672531582950546E-16, -14.41955080893447416, -1.468750000682796708 ) ) ;
#2223=VERTEX_POINT ( 'NONE', #4672 ) ;
#2228=CARTESIAN_POINT ( 'NONE',  ( 1.500000000000000444, -12.13397459621556607, -2.020833334698926897 ) ) ;
#2235=CARTESIAN_POINT ( 'NONE',  ( -4.000000000000000000, -13.00000000000000533, 0.000000000000000000 ) ) ;
#2239=CARTESIAN_POINT ( 'NONE',  ( 8.692241771943169307E-17, -11.58044919106553294, -0.09375000068279677745 ) ) ;
#2241=CARTESIAN_POINT ( 'NONE',  ( 0.000000000000000000, -13.00000000000000533, -3.000000000000000000 ) ) ;
#2244=CARTESIAN_POINT ( 'NONE',  ( -1.500000000000002665, -13.86602540378444282, -2.270833334698926453 ) ) ;
#2252=CARTESIAN_POINT ( 'NONE',  ( -1.500000000000000666, -13.86602540378444459, -1.708333333333333481 ) ) ;
#2259=VERTEX_POINT ( 'NONE', #9013 ) ;
#2279=EDGE_CURVE ( 'NONE', #9635, #6751, #7210, .T. ) ;
#2282=CARTESIAN_POINT ( 'NONE',  ( -0.7500000000000007772, -14.29903810567666156, -0.7291666680322601568 ) ) ;
#2287=CARTESIAN_POINT ( 'NONE',  ( -0.6146835312499998594, -11.93533689329915326, -2.677083334016129967 ) ) ;
#2289=CARTESIAN_POINT ( 'NONE',  ( -2.607672531582950546E-16, -14.41955080893447416, -1.468750000682796708 ) ) ;
#2294=VECTOR ( 'NONE', #9909, 1000.000000000000000 ) ;
#2295=EDGE_LOOP ( 'NONE', ( #2916, #6667, #9251, #5439 ) ) ;
#2301=CARTESIAN_POINT ( 'NONE',  ( -1.500000000000000222, -13.00000000000000533, -1.750000000000000000 ) ) ;
#2308=CARTESIAN_POINT ( 'NONE',  ( -1.500000000000000000, -12.13397459621556607, -2.291666666666666963 ) ) ;
#2309=ORIENTED_EDGE ( 'NONE', *, *, #10325, .T. ) ;
#2311=CARTESIAN_POINT ( 'NONE',  ( 1.500000000000000222, -12.13397459621556784, -0.9583333333333337034 ) ) ;
#2330=CARTESIAN_POINT ( 'NONE',  ( 8.692241771943169307E-17, -11.58044919106553294, -2.593750000682796486 ) ) ;
#2334=CARTESIAN_POINT ( 'NONE',  ( -1.500000000000003775, -13.86602540378444104, -0.7708333346989270085 ) ) ;
#2347=CARTESIAN_POINT ( 'NONE',  ( -1.500000000000000666, -13.86602540378444637, -1.770833334698926897 ) ) ;
#2349=ORIENTED_EDGE ( 'NONE', *, *, #2486, .T. ) ;
#2351=ADVANCED_FACE ( 'NONE', ( #1699 ), #5815, .F. ) ;
#2352=CARTESIAN_POINT ( 'NONE',  ( 1.499999999999999778, -13.86602540378444637, -1.541666666666666963 ) ) ;
#2358=CARTESIAN_POINT ( 'NONE',  ( -0.7500000000000007772, -14.29903810567666156, -2.166666666666666519 ) ) ;
#2372=SURFACE_SIDE_STYLE ('',( #5018 ) ) ;
#2383=CARTESIAN_POINT ( 'NONE',  ( 0.7500000000000003331, -11.70096189432334732, -0.4791666680322602123 ) ) ;
#2389=EDGE_CURVE ( 'NONE', #9588, #4358, #3181, .T. ) ;
#2390=DIRECTION ( 'NONE',  ( -1.000000000000000000, 0.000000000000000000, 0.000000000000000000 ) ) ;
#2399=CARTESIAN_POINT ( 'NONE',  ( 8.692241771943169307E-17, -11.58044919106553294, -1.218750000682796930 ) ) ;
#2417=CARTESIAN_POINT ( 'NONE',  ( -1.500000000000000666, -13.86602540378444459, -0.2083333333333333703 ) ) ;
#2433=CARTESIAN_POINT ( 'NONE',  ( -1.500000000000000222, -13.00000000000000533, -3.000000000000000000 ) ) ;
#2439=CARTESIAN_POINT ( 'NONE',  ( 1.500000000000000222, -13.00000000000000533, -0.06250000136559345776 ) ) ;
#2446=DIRECTION ( 'NONE',  ( -0.8660254037844397068, -0.000000000000000000, 0.4999999999999983347 ) ) ;
#2453=CARTESIAN_POINT ( 'NONE',  ( 0.6146835312500001924, -11.93533689329915326, -0.7604166673494633377 ) ) ;
#2469=CARTESIAN_POINT ( 'NONE',  ( 1.060575238724907038E-16, -11.26794919243112680, -0.3750000000000003886 ) ) ;
#2486=EDGE_CURVE ( 'NONE', #8955, #9594, #5278, .T. ) ;
#2492=CARTESIAN_POINT ( 'NONE',  ( 1.500000000000000444, -12.13397459621556607, -1.020833334698926897 ) ) ;
#2495=CARTESIAN_POINT ( 'NONE',  ( 1.229367062500000163, -13.00000000000000533, 0.2812499993172035695 ) ) ;
#2541=CARTESIAN_POINT ( 'NONE',  ( 1.229367062499999719, -13.70977540446724063, -0.7604166673494633377 ) ) ;
#2551=CARTESIAN_POINT ( 'NONE',  ( 1.229367062500000163, -12.29022459553277002, -1.802083334016129967 ) ) ;
#2581=( BOUNDED_CURVE ( )  B_SPLINE_CURVE ( 2, ( #4447, #279, #6935, #9182, #1972, #10089, #10193, #2709, #2862, #6886, #3504, #2074, #3554 ),
 .UNSPECIFIED., .F., .T. ) 
 B_SPLINE_CURVE_WITH_KNOTS ( ( 3, 2, 2, 2, 2, 2, 3 ),
 ( 0.8538060088535064374, 0.8611111111111111605, 0.8888888888888888395, 0.9166666666666666297, 0.9444444444444444198, 0.9722222222222222099, 1.000000000000000000 ),
 .UNSPECIFIED. ) 
 CURVE ( )  GEOMETRIC_REPRESENTATION_ITEM ( )  RATIONAL_B_SPLINE_CURVE ( ( 0.9480652127606681301, 0.9647668674900647945, 1.000000000000000000, 0.8660254037844387076, 1.000000000000000000, 0.8660254037844387076, 1.000000000000000000, 0.8660254037844387076, 1.000000000000000000, 0.8660254037844387076, 1.000000000000000000, 0.8660254037844387076, 1.000000000000000000 ) ) 
 REPRESENTATION_ITEM ( '' )  );
#2582=FACE_OUTER_BOUND ( 'NONE', #708, .T. ) ;
#2587=LINE ( 'NONE', #4912, #5994 ) ;
#2595=CARTESIAN_POINT ( 'NONE',  ( 8.692241771943169307E-17, -11.58044919106553294, -1.093750000682796486 ) ) ;
#2598=EDGE_LOOP ( 'NONE', ( #5762, #1261, #3804, #1806 ) ) ;
#2605=CARTESIAN_POINT ( 'NONE',  ( 0.6146835312499993043, -14.06466310670085562, -1.927083334016129967 ) ) ;
#2607=EDGE_CURVE ( 'NONE', #9521, #8600, #1543, .T. ) ;
#2612=CARTESIAN_POINT ( 'NONE',  ( 0.000000000000000000, -13.00000000000000533, 0.000000000000000000 ) ) ;
#2619=CARTESIAN_POINT ( 'NONE',  ( -1.229367062500000163, -13.00000000000000533, -2.468750000682796486 ) ) ;
#2627=EDGE_LOOP ( 'NONE', ( #6418, #4531, #6663, #339 ) ) ;
#2629=DIRECTION ( 'NONE',  ( -0.000000000000000000, -0.000000000000000000, -1.000000000000000000 ) ) ;
#2630=ORIENTED_EDGE ( 'NONE', *, *, #9628, .F. ) ;
#2632=CARTESIAN_POINT ( 'NONE',  ( 8.692241771943169307E-17, -11.58044919106553294, -2.718750000682796042 ) ) ;
#2641=ADVANCED_FACE ( 'NONE', ( #3893 ), #9530, .T. ) ;
#2646=CARTESIAN_POINT ( 'NONE',  ( -1.229367062500000385, -13.70977540446723886, -0.4270833340161298564 ) ) ;
#2655=CARTESIAN_POINT ( 'NONE',  ( 1.229367062500000163, -13.00000000000000533, -1.843750000682796708 ) ) ;
#2667=CARTESIAN_POINT ( 'NONE',  ( 0.6146835312499993043, -14.06466310670085562, -1.302083334016129967 ) ) ;
#2678=EDGE_CURVE ( 'NONE', #1372, #274, #2849, .T. ) ;
#2687=ORIENTED_EDGE ( 'NONE', *, *, #5598, .T. ) ;
#2692=CARTESIAN_POINT ( 'NONE',  ( -0.6146835312499998594, -11.93533689329915326, -2.052083334016129967 ) ) ;
#2700=AXIS2_PLACEMENT_3D ( 'NONE', #3352, #3198, #6422 ) ;
#2701=CARTESIAN_POINT ( 'NONE',  ( 1.229367062500000163, -12.29022459553277002, -2.302083334016129967 ) ) ;
#2709=CARTESIAN_POINT ( 'NONE',  ( -1.500000000000000666, -13.86602540378444637, 0.2291666653010732135 ) ) ;
#2715=DIRECTION ( 'NONE',  ( 0.000000000000000000, 0.000000000000000000, 1.000000000000000000 ) ) ;
#2723=ORIENTED_EDGE ( 'NONE', *, *, #6351, .T. ) ;
#2737=CARTESIAN_POINT ( 'NONE',  ( -0.6146835312500006365, -14.06466310670085562, -2.510416667349463005 ) ) ;
#2741=CARTESIAN_POINT ( 'NONE',  ( 0.7499999999999991118, -14.29903810567666333, -0.5833333333333332593 ) ) ;
#2749=CARTESIAN_POINT ( 'NONE',  ( -1.229367062500000163, -12.29022459553277002, -2.010416667349463005 ) ) ;
#2756=CARTESIAN_POINT ( 'NONE',  ( 1.229367062500000163, -13.70977540446723886, -1.885416667349463449 ) ) ;
#2768=DIRECTION ( 'NONE',  ( 0.000000000000000000, -1.000000000000000000, 0.000000000000000000 ) ) ;
#2770=CARTESIAN_POINT ( 'NONE',  ( 1.229367062500000163, -13.00000000000000533, -2.218750000682796486 ) ) ;
#2773=CARTESIAN_POINT ( 'NONE',  ( -0.6146835312499998594, -11.93533689329915326, -0.05208333401612993963 ) ) ;
#2784=CARTESIAN_POINT ( 'NONE',  ( -2.607672531582950546E-16, -14.41955080893447416, -0.9687500006827967081 ) ) ;
#2788=CARTESIAN_POINT ( 'NONE',  ( -3.181725716174720991E-16, -14.73205080756888563, -0.6250000000000001110 ) ) ;
#2817=CARTESIAN_POINT ( 'NONE',  ( 0.7499999999999991118, -14.29903810567666333, -0.08333333333333370341 ) ) ;
#2821=CARTESIAN_POINT ( 'NONE',  ( -4.000000000000000000, -13.00000000000000533, 2.000000000000000000 ) ) ;
#2823=CARTESIAN_POINT ( 'NONE',  ( 0.6146835312500001924, -11.93533689329915326, -1.635416667349463227 ) ) ;
#2825=CARTESIAN_POINT ( 'NONE',  ( -1.229367062500000163, -12.29022459553277002, -0.01041666734946308792 ) ) ;
#2831=ORIENTED_EDGE ( 'NONE', *, *, #7501, .F. ) ;
#2834=CARTESIAN_POINT ( 'NONE',  ( 0.6146835312500001924, -11.93533689329915326, -1.260416667349463227 ) ) ;
#2838=CARTESIAN_POINT ( 'NONE',  ( -1.500000000000000222, -13.00000000000000533, -0.7500000000000002220 ) ) ;
#2841=EDGE_LOOP ( 'NONE', ( #560, #5127 ) ) ;
#2849=( BOUNDED_CURVE ( )  B_SPLINE_CURVE ( 2, ( #5585, #2311, #7875, #5481, #5534, #7988, #4007 ),
 .UNSPECIFIED., .F., .F. ) 
 B_SPLINE_CURVE_WITH_KNOTS ( ( 3, 2, 2, 3 ),
 ( 0.6666666666666666297, 0.6944444444444444198, 0.7222222222222222099, 0.7500000000000000000 ),
 .UNSPECIFIED. ) 
 CURVE ( )  GEOMETRIC_REPRESENTATION_ITEM ( )  RATIONAL_B_SPLINE_CURVE ( ( 1.000000000000000000, 0.8660254037844387076, 1.000000000000000000, 0.8660254037844387076, 1.000000000000000000, 0.8660254037844387076, 1.000000000000000000 ) ) 
 REPRESENTATION_ITEM ( '' )  );
#2858=CARTESIAN_POINT ( 'NONE',  ( -1.500000000000000666, -13.86602540378444459, -2.270833334698926453 ) ) ;
#2862=CARTESIAN_POINT ( 'NONE',  ( -0.7500000000000007772, -14.29903810567666156, 0.2708333319677396211 ) ) ;
#2870=CARTESIAN_POINT ( 'NONE',  ( -1.229367062500000385, -13.70977540446723886, -2.052083334016129967 ) ) ;
#2873=CARTESIAN_POINT ( 'NONE',  ( 1.229367062500000163, -12.29022459553277002, -1.677083334016129967 ) ) ;
#2887=CARTESIAN_POINT ( 'NONE',  ( -1.500000000000000000, -12.13397459621556607, -2.791666666666666519 ) ) ;
#2916=ORIENTED_EDGE ( 'NONE', *, *, #7531, .F. ) ;
#2917=CARTESIAN_POINT ( 'NONE',  ( 1.500000000000000222, -13.00000000000000533, -2.062500001365593416 ) ) ;
#2918=CARTESIAN_POINT ( 'NONE',  ( -1.499999999999999778, -12.13397459621556784, -0.3541666680322601013 ) ) ;
#2919=( BOUNDED_CURVE ( )  B_SPLINE_CURVE ( 2, ( #6653, #4319, #4966, #7463, #3377, #5803, #1095 ),
 .UNSPECIFIED., .F., .T. ) 
 B_SPLINE_CURVE_WITH_KNOTS ( ( 3, 2, 2, 3 ),
 ( 0.8333333333333332593, 0.8611111111111110494, 0.8888888888888888395, 0.9166666666666666297 ),
 .UNSPECIFIED. ) 
 CURVE ( )  GEOMETRIC_REPRESENTATION_ITEM ( )  RATIONAL_B_SPLINE_CURVE ( ( 1.000000000000000444, 0.8660254037844381525, 1.000000000000000000, 0.8660254037844387076, 1.000000000000000000, 0.8660254037844387076, 1.000000000000000000 ) ) 
 REPRESENTATION_ITEM ( '' )  );
#2928=CARTESIAN_POINT ( 'NONE',  ( -2.607672531582950546E-16, -14.41955080893447416, -0.3437500006827965415 ) ) ;
#2930=CARTESIAN_POINT ( 'NONE',  ( 1.229367062500000163, -13.00000000000000533, 0.2812499993172035695 ) ) ;
#2944=CARTESIAN_POINT ( 'NONE',  ( 1.229367062499999719, -13.70977540446724063, -1.885416667349463449 ) ) ;
#2954=ORIENTED_EDGE ( 'NONE', *, *, #8671, .F. ) ;
#2955=CARTESIAN_POINT ( 'NONE',  ( 1.060575238724907038E-16, -11.26794919243112680, -1.437500001365593416 ) ) ;
#2967=ORIENTED_EDGE ( 'NONE', *, *, #8249, .F. ) ;
#2981=CARTESIAN_POINT ( 'NONE',  ( -2.607672531582950546E-16, -14.41955080893447416, 0.1562499993172034585 ) ) ;
#2991=LINE ( 'NONE', #4620, #5759 ) ;
#2997=CARTESIAN_POINT ( 'NONE',  ( -3.181725716174720498E-16, -14.73205080756888385, -2.625000000000000000 ) ) ;
#3007=CARTESIAN_POINT ( 'NONE',  ( -0.7499999999999997780, -11.70096189432334555, -1.395833334698926897 ) ) ;
#3016=CARTESIAN_POINT ( 'NONE',  ( 1.364683531250000303, -13.00000000000000533, 0.07812499965860171536 ) ) ;
#3018=ORIENTED_EDGE ( 'NONE', *, *, #859, .F. ) ;
#3029=CARTESIAN_POINT ( 'NONE',  ( -1.229367062500000163, -13.00000000000000533, -2.093750000682796930 ) ) ;
#3048=CARTESIAN_POINT ( 'NONE',  ( 1.500000000000000222, -13.00000000000000533, -2.500000000000000000 ) ) ;
#3051=CARTESIAN_POINT ( 'NONE',  ( 0.000000000000000000, -13.00000000000000533, -3.000000000000000000 ) ) ;
#3059=ORIENTED_EDGE ( 'NONE', *, *, #7, .T. ) ;
#3062=VECTOR ( 'NONE', #7711, 1000.000000000000000 ) ;
#3073=CARTESIAN_POINT ( 'NONE',  ( -1.500000000000000222, -13.00000000000000533, -2.312500001365593860 ) ) ;
#3083=CARTESIAN_POINT ( 'NONE',  ( -1.229367062500000163, -13.00000000000000533, -0.4687500006827967081 ) ) ;
#3095=FILL_AREA_STYLE ('',( #9575 ) ) ;
#3099=CARTESIAN_POINT ( 'NONE',  ( 1.500000000000000000, -13.86602540378444459, -2.041666666666666963 ) ) ;
#3122=CARTESIAN_POINT ( 'NONE',  ( -0.7500000000000007772, -14.29903810567666156, -1.229166668032260157 ) ) ;
#3129=CARTESIAN_POINT ( 'NONE',  ( -0.7499999999999997780, -11.70096189432334555, -2.333333333333333481 ) ) ;
#3134=CARTESIAN_POINT ( 'NONE',  ( -1.229367062500000385, -13.70977540446723886, -1.052083334016129967 ) ) ;
#3153=CARTESIAN_POINT ( 'NONE',  ( -0.7499999999999997780, -11.70096189432334555, -2.333333333333333481 ) ) ;
#3168=DIRECTION ( 'NONE',  ( 0.000000000000000000, 0.000000000000000000, 1.000000000000000000 ) ) ;
#3174=CARTESIAN_POINT ( 'NONE',  ( -3.181725716174720498E-16, -14.73205080756888385, -1.687500001365593638 ) ) ;
#3176=CARTESIAN_POINT ( 'NONE',  ( -1.500000000000000222, -13.00000000000000533, -1.312500001365593416 ) ) ;
#3181=LINE ( 'NONE', #9768, #7297 ) ;
#3188=ADVANCED_FACE ( 'NONE', ( #8762 ), #3196, .T. ) ;
#3189=CARTESIAN_POINT ( 'NONE',  ( 1.229367062499999719, -13.70977540446724063, -0.8854166673494634487 ) ) ;
#3196=CYLINDRICAL_SURFACE ( 'NONE', #6525, 1.500000000000000222 ) ;
#3198=DIRECTION ( 'NONE',  ( 0.000000000000000000, 0.000000000000000000, 1.000000000000000000 ) ) ;
#3203=CARTESIAN_POINT ( 'NONE',  ( -1.500000000000000222, -13.00000000000000533, -1.250000000000000000 ) ) ;
#3215=SURFACE_STYLE_USAGE ( .BOTH. , #2372 ) ;
#3216=VECTOR ( 'NONE', #1587, 1000.000000000000000 ) ;
#3226=CARTESIAN_POINT ( 'NONE',  ( 1.060575238724907038E-16, -11.26794919243112680, -0.4375000013655937492 ) ) ;
#3249=CARTESIAN_POINT ( 'NONE',  ( 0.7499999999999991118, -14.29903810567666333, -1.645833334698926675 ) ) ;
#3250=CARTESIAN_POINT ( 'NONE',  ( 1.500000000000000222, -13.00000000000000533, -0.06250000136559345776 ) ) ;
#3257=CARTESIAN_POINT ( 'NONE',  ( 0.7499999999999991118, -14.29903810567666333, -0.5833333333333332593 ) ) ;
#3260=( BOUNDED_CURVE ( )  B_SPLINE_CURVE ( 2, ( #7762, #8767, #1506, #7867, #5419, #9464, #10426 ),
 .UNSPECIFIED., .F., .T. ) 
 B_SPLINE_CURVE_WITH_KNOTS ( ( 3, 2, 2, 3 ),
 ( 0.7500000000000000000, 0.7777777777777777901, 0.8055555555555554692, 0.8333333333333332593 ),
 .UNSPECIFIED. ) 
 CURVE ( )  GEOMETRIC_REPRESENTATION_ITEM ( )  RATIONAL_B_SPLINE_CURVE ( ( 1.000000000000000000, 0.8660254037844387076, 1.000000000000000000, 0.8660254037844387076, 1.000000000000000000, 0.8660254037844392627, 0.9999999999999994449 ) ) 
 REPRESENTATION_ITEM ( '' )  );
#3265=ORIENTED_EDGE ( 'NONE', *, *, #1899, .T. ) ;
#3273=EDGE_LOOP ( 'NONE', ( #3372, #9099, #9711, #958 ) ) ;
#3282=CARTESIAN_POINT ( 'NONE',  ( 1.500000000000000000, -13.86602540378444459, -0.6041666680322602678 ) ) ;
#3285=CARTESIAN_POINT ( 'NONE',  ( -3.181725716174720991E-16, -14.73205080756888563, -2.624999999999999556 ) ) ;
#3292=CARTESIAN_POINT ( 'NONE',  ( 8.692241771943169307E-17, -11.58044919106553294, -0.2187500006827968746 ) ) ;
#3309=CARTESIAN_POINT ( 'NONE',  ( 1.229367062500000163, -13.00000000000000533, -2.718750000682796486 ) ) ;
#3334=CARTESIAN_POINT ( 'NONE',  ( -3.181725716174720498E-16, -14.73205080756888385, -0.1875000013655935549 ) ) ;
#3338=DIRECTION ( 'NONE',  ( 1.000000000000000000, 0.000000000000000000, 0.000000000000000000 ) ) ;
#3340=CARTESIAN_POINT ( 'NONE',  ( 8.692241771943170539E-17, -11.58044919106553650, -2.718750000682796042 ) ) ;
#3349=CARTESIAN_POINT ( 'NONE',  ( 1.499999999999999778, -13.86602540378444637, -1.604166668032260379 ) ) ;
#3352=CARTESIAN_POINT ( 'NONE',  ( 0.000000000000000000, -13.00000000000000533, -3.000000000000000000 ) ) ;
#3370=CARTESIAN_POINT ( 'NONE',  ( -3.181725716174720991E-16, -14.73205080756888563, -1.187500001365593638 ) ) ;
#3372=ORIENTED_EDGE ( 'NONE', *, *, #7501, .T. ) ;
#3374=LINE ( 'NONE', #4170, #3989 ) ;
#3375=EDGE_CURVE ( 'NONE', #6225, #8892, #10460, .T. ) ;
#3377=CARTESIAN_POINT ( 'NONE',  ( -0.7499999999999997780, -11.70096189432334555, -0.3333333333333334814 ) ) ;
#3385=CARTESIAN_POINT ( 'NONE',  ( 1.229367062500000385, -12.29022459553277002, -2.177083334016129523 ) ) ;
#3395=CARTESIAN_POINT ( 'NONE',  ( -2.607672531582950546E-16, -14.41955080893447416, -1.468750000682796708 ) ) ;
#3403=FACE_BOUND ( 'NONE', #7993, .T. ) ;
#3405=ADVANCED_FACE ( 'NONE', ( #1017 ), #4942, .T. ) ;
#3411=LINE ( 'NONE', #3560, #260 ) ;
#3430=CARTESIAN_POINT ( 'NONE',  ( 0.000000000000000000, -13.00000000000000533, -3.000000000000000000 ) ) ;
#3436=CARTESIAN_POINT ( 'NONE',  ( 1.229367062500000163, -13.00000000000000533, -0.2187500006827964583 ) ) ;
#3447=CARTESIAN_POINT ( 'NONE',  ( -2.607672531582950546E-16, -14.41955080893447416, -1.968750000682796708 ) ) ;
#3465=CARTESIAN_POINT ( 'NONE',  ( 0.6146835312500001924, -11.93533689329915326, -2.635416667349463449 ) ) ;
#3482=FACE_OUTER_BOUND ( 'NONE', #9007, .T. ) ;
#3490=CARTESIAN_POINT ( 'NONE',  ( -0.6146835312500006365, -14.06466310670085562, 0.1145833326505365929 ) ) ;
#3494=CARTESIAN_POINT ( 'NONE',  ( 0.000000000000000000, -13.00000000000000533, -3.000000000000000000 ) ) ;
#3499=CARTESIAN_POINT ( 'NONE',  ( -1.229367062500000163, -13.70977540446723708, -0.5520833340161299674 ) ) ;
#3504=CARTESIAN_POINT ( 'NONE',  ( 0.7499999999999991118, -14.29903810567666333, 0.3541666653010728805 ) ) ;
#3507=EDGE_CURVE ( 'NONE', #4078, #2259, #1427, .T. ) ;
#3512=CARTESIAN_POINT ( 'NONE',  ( -1.229367062500000385, -13.70977540446723886, -1.427083334016129745 ) ) ;
#3514=CARTESIAN_POINT ( 'NONE',  ( 0.6146835312500001924, -11.93533689329915326, -2.135416667349463449 ) ) ;
#3523=CARTESIAN_POINT ( 'NONE',  ( -2.607672531582950546E-16, -14.41955080893447416, -2.468750000682796486 ) ) ;
#3530=ORIENTED_EDGE ( 'NONE', *, *, #8031, .F. ) ;
#3536=CARTESIAN_POINT ( 'NONE',  ( -0.6146835312499998594, -11.93533689329915326, -1.552083334016129967 ) ) ;
#3544=AXIS2_PLACEMENT_3D ( 'NONE', #4196, #2768, #8345 ) ;
#3545=CARTESIAN_POINT ( 'NONE',  ( 1.500000000000000222, -13.00000000000000533, -2.562500001365593416 ) ) ;
#3546=CARTESIAN_POINT ( 'NONE',  ( 8.692241771943170539E-17, -11.58044919106553650, -0.2187500006827969301 ) ) ;
#3554=CARTESIAN_POINT ( 'NONE',  ( 1.500000000000000222, -13.00000000000000533, 0.4374999986344065284 ) ) ;
#3560=CARTESIAN_POINT ( 'NONE',  ( -1.500000000000000222, -13.00000000000000533, -3.000000000000000000 ) ) ;
#3562=CARTESIAN_POINT ( 'NONE',  ( -1.229367062500000163, -13.00000000000000533, -0.9687500006827964860 ) ) ;
#3565=CARTESIAN_POINT ( 'NONE',  ( -0.6146835312499998594, -11.93533689329915326, -0.5520833340161299674 ) ) ;
#3578=CARTESIAN_POINT ( 'NONE',  ( -1.229367062500000163, -12.29022459553277002, -1.635416667349463227 ) ) ;
#3590=CARTESIAN_POINT ( 'NONE',  ( -1.229367062500000163, -12.29022459553277002, -0.5104166673494631157 ) ) ;
#3598=CARTESIAN_POINT ( 'NONE',  ( 1.070288219556879694, -11.94905607805280567, 1.518836458664385706E-16 ) ) ;
#3612=CARTESIAN_POINT ( 'NONE',  ( 1.229367062500000385, -12.29022459553277002, -2.177083334016129523 ) ) ;
#3615=CARTESIAN_POINT ( 'NONE',  ( -1.229367062500000163, -12.29022459553277002, -2.010416667349463005 ) ) ;
#3626=CARTESIAN_POINT ( 'NONE',  ( 1.500000000000000222, -13.00000000000000533, -3.000000000000000000 ) ) ;
#3660=DIRECTION ( 'NONE',  ( 0.000000000000000000, 0.000000000000000000, 1.000000000000000000 ) ) ;
#3665=CARTESIAN_POINT ( 'NONE',  ( -0.6146835312500006365, -14.06466310670085562, -1.885416667349463227 ) ) ;
#3679=CARTESIAN_POINT ( 'NONE',  ( 1.060575238724907038E-16, -11.26794919243112680, -2.875000000000000000 ) ) ;
#3698=PLANE ( 'NONE',  #6668 ) ;
#3701=CARTESIAN_POINT ( 'NONE',  ( -1.500000000000000000, -12.13397459621556607, -2.354166668032260379 ) ) ;
#3714=CARTESIAN_POINT ( 'NONE',  ( 1.229367062500000163, -13.00000000000000533, -1.843750000682796708 ) ) ;
#3717=CARTESIAN_POINT ( 'NONE',  ( 1.229367062500000163, -12.29022459553277002, -0.6770833340161300784 ) ) ;
#3730=CARTESIAN_POINT ( 'NONE',  ( -0.6146835312500006365, -14.06466310670085562, -1.510416667349463227 ) ) ;
#3732=VECTOR ( 'NONE', #2446, 999.9999999999998863 ) ;
#3735=CARTESIAN_POINT ( 'NONE',  ( 0.000000000000000000, -13.00000000000000533, -3.000000000000000000 ) ) ;
#3743=CARTESIAN_POINT ( 'NONE',  ( -1.500000000000000222, -13.00000000000000533, -1.250000000000000000 ) ) ;
#3767=CARTESIAN_POINT ( 'NONE',  ( 0.6146835312500001924, -11.93533689329915326, -1.760416667349463449 ) ) ;
#3769=CARTESIAN_POINT ( 'NONE',  ( -1.229367062500000163, -13.70977540446723708, -1.927083334016129745 ) ) ;
#3782=CARTESIAN_POINT ( 'NONE',  ( 1.229367062500000163, -13.00000000000000533, -0.8437500006827965970 ) ) ;
#3800=ORIENTED_EDGE ( 'NONE', *, *, #1033, .F. ) ;
#3802=CARTESIAN_POINT ( 'NONE',  ( -1.500000000000000222, -13.00000000000000533, -1.312500001365593416 ) ) ;
#3804=ORIENTED_EDGE ( 'NONE', *, *, #5876, .T. ) ;
#3812=EDGE_CURVE ( 'NONE', #9003, #1372, #7185, .T. ) ;
#3819=CARTESIAN_POINT ( 'NONE',  ( -0.6146835312499998594, -11.93533689329915326, -0.5520833340161299674 ) ) ;
#3831=CARTESIAN_POINT ( 'NONE',  ( -3.181725716174720991E-16, -14.73205080756888563, -1.625000000000000222 ) ) ;
#3836=CARTESIAN_POINT ( 'NONE',  ( 1.060575238724907038E-16, -11.26794919243112680, -1.875000000000000222 ) ) ;
#3844=LINE ( 'NONE', #8723, #829 ) ;
#3847=CARTESIAN_POINT ( 'NONE',  ( 1.500000000000000222, -12.13397459621556784, -1.520833334698926897 ) ) ;
#3859=ORIENTED_EDGE ( 'NONE', *, *, #6829, .F. ) ;
#3860=CARTESIAN_POINT ( 'NONE',  ( -0.7499999999999997780, -11.70096189432334555, -1.895833334698926897 ) ) ;
#3861=CARTESIAN_POINT ( 'NONE',  ( 1.500000000000000222, -12.13397459621556784, -0.5208333346989270085 ) ) ;
#3865=CARTESIAN_POINT ( 'NONE',  ( -1.500000000000000222, -13.00000000000000533, -2.250000000000000444 ) ) ;
#3870=CARTESIAN_POINT ( 'NONE',  ( -1.229367062500000385, -13.70977540446723886, -2.552083334016129967 ) ) ;
#3881=LINE ( 'NONE', #10481, #1195 ) ;
#3889=CARTESIAN_POINT ( 'NONE',  ( 1.500000000000000444, -12.13397459621556607, -1.458333333333333481 ) ) ;
#3893=FACE_OUTER_BOUND ( 'NONE', #367, .T. ) ;
#3895=CARTESIAN_POINT ( 'NONE',  ( -1.499999999999997780, -12.13397459621556429, -2.354166668032259935 ) ) ;
#3898=LINE ( 'NONE', #1576, #7431 ) ;
#3918=CARTESIAN_POINT ( 'NONE',  ( -1.500000000000000666, -13.86602540378444459, 0.2291666653010731858 ) ) ;
#3936=( BOUNDED_CURVE ( )  B_SPLINE_CURVE ( 2, ( #4587, #564, #8526, #9374, #2006, #8675, #3743 ),
 .UNSPECIFIED., .F., .T. ) 
 B_SPLINE_CURVE_WITH_KNOTS ( ( 3, 2, 2, 3 ),
 ( 0.5000000000000000000, 0.5277777777777777901, 0.5555555555555554692, 0.5833333333333332593 ),
 .UNSPECIFIED. ) 
 CURVE ( )  GEOMETRIC_REPRESENTATION_ITEM ( )  RATIONAL_B_SPLINE_CURVE ( ( 1.000000000000000000, 0.8660254037844387076, 1.000000000000000000, 0.8660254037844387076, 1.000000000000000000, 0.8660254037844392627, 0.9999999999999994449 ) ) 
 REPRESENTATION_ITEM ( '' )  );
#3940=CARTESIAN_POINT ( 'NONE',  ( 0.000000000000000000, -13.00000000000000533, -3.000000000000000000 ) ) ;
#3945=CARTESIAN_POINT ( 'NONE',  ( 1.500000000000000000, -13.86602540378444459, -2.541666666666666963 ) ) ;
#3953=DIRECTION ( 'NONE',  ( 1.000000000000000000, 0.000000000000000000, 0.000000000000000000 ) ) ;
#3964=ADVANCED_FACE ( 'NONE', ( #6567 ), #4932, .F. ) ;
#3972=CARTESIAN_POINT ( 'NONE',  ( 1.060575238724907038E-16, -11.26794919243112680, -1.437500001365593416 ) ) ;
#3977=FACE_OUTER_BOUND ( 'NONE', #5477, .T. ) ;
#3981=AXIS2_PLACEMENT_3D ( 'NONE', #3494, #1698, #217 ) ;
#3988=DIRECTION ( 'NONE',  ( 1.000000000000000000, 0.000000000000000000, 0.000000000000000000 ) ) ;
#3989=VECTOR ( 'NONE', #4859, 1000.000000000000000 ) ;
#4004=CARTESIAN_POINT ( 'NONE',  ( -1.500000000000000666, -13.86602540378444459, -0.7083333333333333703 ) ) ;
#4007=CARTESIAN_POINT ( 'NONE',  ( -1.500000000000000222, -13.00000000000000533, -0.7500000000000002220 ) ) ;
#4016=ORIENTED_EDGE ( 'NONE', *, *, #7981, .T. ) ;
#4018=CARTESIAN_POINT ( 'NONE',  ( -1.500000000000000222, -13.00000000000000533, -1.750000000000000000 ) ) ;
#4024=CARTESIAN_POINT ( 'NONE',  ( -3.181725716174720498E-16, -14.73205080756888385, -0.6875000013655935271 ) ) ;
#4029=CARTESIAN_POINT ( 'NONE',  ( 0.7499999999999991118, -14.29903810567666333, -2.083333333333333481 ) ) ;
#4049=CARTESIAN_POINT ( 'NONE',  ( -1.500000000000000000, -12.13397459621556607, -0.7916666666666666297 ) ) ;
#4051=ORIENTED_EDGE ( 'NONE', *, *, #7, .F. ) ;
#4069=ORIENTED_EDGE ( 'NONE', *, *, #6660, .F. ) ;
#4075=CARTESIAN_POINT ( 'NONE',  ( -1.500000000000000222, -13.00000000000000533, 0.1874999986344063341 ) ) ;
#4078=VERTEX_POINT ( 'NONE', #9175 ) ;
#4089=CARTESIAN_POINT ( 'NONE',  ( -1.229367062500000385, -13.70977540446723886, -0.5520833340161299674 ) ) ;
#4124=CARTESIAN_POINT ( 'NONE',  ( 1.500000000000000000, -13.86602540378444459, -1.104166668032260379 ) ) ;
#4128=CARTESIAN_POINT ( 'NONE',  ( 1.364683531250000303, -13.00000000000000533, 0.07812499965860171536 ) ) ;
#4131=DIRECTION ( 'NONE',  ( 1.000000000000000000, 0.000000000000000000, -0.000000000000000000 ) ) ;
#4136=CARTESIAN_POINT ( 'NONE',  ( 8.692241771943169307E-17, -11.58044919106553294, -0.7187500006827969301 ) ) ;
#4147=DIRECTION ( 'NONE',  ( 0.000000000000000000, 0.000000000000000000, 1.000000000000000000 ) ) ;
#4160=EDGE_LOOP ( 'NONE', ( #9061, #9473, #6603 ) ) ;
#4166=CARTESIAN_POINT ( 'NONE',  ( 0.7499999999999991118, -14.29903810567666333, -1.145833334698926897 ) ) ;
#4170=CARTESIAN_POINT ( 'NONE',  ( 1.500000000000000222, -13.00000000000000533, -2.781250000682796486 ) ) ;
#4177=CARTESIAN_POINT ( 'NONE',  ( 1.229367062500000385, -12.29022459553277002, -1.677083334016129967 ) ) ;
#4186=CARTESIAN_POINT ( 'NONE',  ( 1.229367062500000163, -13.70977540446723886, -0.8854166673494634487 ) ) ;
#4196=CARTESIAN_POINT ( 'NONE',  ( 1.364683531250000303, -13.00000000000000533, -2.921875000341398465 ) ) ;
#4208=CARTESIAN_POINT ( 'NONE',  ( 1.500000000000000222, -13.00000000000000533, 0.2187499993172032642 ) ) ;
#4216=DIRECTION ( 'NONE',  ( -0.000000000000000000, -0.000000000000000000, -1.000000000000000000 ) ) ;
#4226=ORIENTED_EDGE ( 'NONE', *, *, #2678, .T. ) ;
#4227=CARTESIAN_POINT ( 'NONE',  ( -1.229367062500000163, -13.00000000000000533, -1.968750000682796708 ) ) ;
#4231=CARTESIAN_POINT ( 'NONE',  ( -1.500000000000000222, -13.00000000000000533, -3.000000000000000000 ) ) ;
#4236=CARTESIAN_POINT ( 'NONE',  ( -0.6146835312499998594, -11.93533689329915326, -0.6770833340161300784 ) ) ;
#4245=CARTESIAN_POINT ( 'NONE',  ( 0.000000000000000000, -13.00000000000000533, -3.000000000000000000 ) ) ;
#4249=CARTESIAN_POINT ( 'NONE',  ( 1.229367062500000163, -13.00000000000000533, -1.718750000682796486 ) ) ;
#4251=CARTESIAN_POINT ( 'NONE',  ( -1.229367062500000163, -12.29022459553277002, -2.510416667349463449 ) ) ;
#4270=( BOUNDED_CURVE ( )  B_SPLINE_CURVE ( 2, ( #8175, #907, #116, #3340, #2287, #374, #6772, #1860, #1755, #9875, #4286, #9017, #1914, #2701, #6568, #10035, #8228, #6670, #1112, #4982, #7482, #3447, #2605, #2756, #2655, #2551, #7527, #9928, #5920, #5768, #1160, #5869, #5821, #3395, #960, #5034, #4387, #6624, #9074, #7633, #9819, #1808, #8280, #222, #6716, #9176, #9120, #4186, #1006, #5083, #8336, #4337, #4236, #1063, #272, #3499, #9976, #320, #7420, #5136, #163, #8382, #7577, #3546, #5971, #9225, #1965, #5187, #8434, #1465, #7991, #6278, #5293 ),
 .UNSPECIFIED., .F., .T. ) 
 B_SPLINE_CURVE_WITH_KNOTS ( ( 3, 2, 2, 2, 2, 2, 2, 2, 2, 2, 2, 2, 2, 2, 2, 2, 2, 2, 2, 2, 2, 2, 2, 2, 2, 2, 2, 2, 2, 2, 2, 2, 2, 2, 2, 2, 3 ),
 ( 0.000000000000000000, 0.02777777777777777624, 0.05555555555555555247, 0.08333333333333332871, 0.1111111111111111049, 0.1388888888888888951, 0.1666666666666666574, 0.1944444444444444475, 0.2222222222222222099, 0.2500000000000000000, 0.2777777777777777901, 0.3055555555555555802, 0.3333333333333333148, 0.3611111111111111049, 0.3888888888888888951, 0.4166666666666666852, 0.4444444444444444198, 0.4722222222222222099, 0.5000000000000000000, 0.5277777777777777901, 0.5555555555555555802, 0.5833333333333333703, 0.6111111111111111605, 0.6388888888888888395, 0.6666666666666666297, 0.6944444444444444198, 0.7222222222222222099, 0.7500000000000000000, 0.7777777777777777901, 0.8055555555555555802, 0.8333333333333333703, 0.8611111111111111605, 0.8888888888888888395, 0.9166666666666666297, 0.9444444444444444198, 0.9722222222222222099, 1.000000000000000000 ),
 .UNSPECIFIED. ) 
 CURVE ( )  GEOMETRIC_REPRESENTATION_ITEM ( )  RATIONAL_B_SPLINE_CURVE ( ( 1.000000000000000000, 0.8660254037844387076, 1.000000000000000000, 0.8660254037844387076, 1.000000000000000000, 0.8660254037844387076, 1.000000000000000000, 0.8660254037844387076, 1.000000000000000000, 0.8660254037844387076, 1.000000000000000000, 0.8660254037844387076, 1.000000000000000000, 0.8660254037844387076, 1.000000000000000000, 0.8660254037844387076, 1.000000000000000000, 0.8660254037844387076, 1.000000000000000000, 0.8660254037844387076, 1.000000000000000000, 0.8660254037844387076, 1.000000000000000000, 0.8660254037844387076, 1.000000000000000000, 0.8660254037844387076, 1.000000000000000000, 0.8660254037844387076, 1.000000000000000000, 0.8660254037844387076, 1.000000000000000000, 0.8660254037844387076, 1.000000000000000000, 0.8660254037844387076, 1.000000000000000000, 0.8660254037844387076, 1.000000000000000000, 0.8660254037844387076, 1.000000000000000000, 0.8660254037844387076, 1.000000000000000000, 0.8660254037844387076, 1.000000000000000000, 0.8660254037844387076, 1.000000000000000000, 0.8660254037844387076, 1.000000000000000000, 0.8660254037844387076, 1.000000000000000000, 0.8660254037844387076, 1.000000000000000000, 0.8660254037844387076, 1.000000000000000000, 0.8660254037844387076, 1.000000000000000000, 0.8660254037844387076, 1.000000000000000000, 0.8660254037844387076, 1.000000000000000000, 0.8660254037844387076, 1.000000000000000000, 0.8660254037844387076, 1.000000000000000000, 0.8660254037844387076, 1.000000000000000000, 0.8660254037844387076, 1.000000000000000000, 0.8660254037844387076, 1.000000000000000000, 0.8660254037844387076, 1.000000000000000000, 0.8660254037844387076, 1.000000000000000000 ) ) 
 REPRESENTATION_ITEM ( '' )  );
#4275=CARTESIAN_POINT ( 'NONE',  ( 0.6146835312500001924, -11.93533689329915326, -0.1354166673494631989 ) ) ;
#4286=CARTESIAN_POINT ( 'NONE',  ( 0.6146835312499993043, -14.06466310670085562, -2.427083334016129967 ) ) ;
#4298=CARTESIAN_POINT ( 'NONE',  ( -1.229367062500000163, -13.00000000000000533, -1.968750000682796708 ) ) ;
#4301=CARTESIAN_POINT ( 'NONE',  ( 1.229367062500000163, -12.29022459553277002, -2.677083334016129079 ) ) ;
#4312=CARTESIAN_POINT ( 'NONE',  ( 0.6146835312500001924, -11.93533689329915326, -2.760416667349463449 ) ) ;
#4319=CARTESIAN_POINT ( 'NONE',  ( 1.500000000000003775, -12.13397459621556962, -0.4583333333333337034 ) ) ;
#4324=ORIENTED_EDGE ( 'NONE', *, *, #343, .F. ) ;
#4326=CARTESIAN_POINT ( 'NONE',  ( 0.6146835312499993043, -14.06466310670085562, -0.3020833340161297453 ) ) ;
#4331=( BOUNDED_CURVE ( )  B_SPLINE_CURVE ( 2, ( #8720, #775, #7069, #6217, #10318, #3895, #5433 ),
 .UNSPECIFIED., .F., .F. ) 
 B_SPLINE_CURVE_WITH_KNOTS ( ( 3, 2, 2, 3 ),
 ( 0.000000000000000000, 0.02777777777777775195, 0.05555555555555550390, 0.08333333333333325932 ),
 .UNSPECIFIED. ) 
 CURVE ( )  GEOMETRIC_REPRESENTATION_ITEM ( )  RATIONAL_B_SPLINE_CURVE ( ( 1.000000000000000000, 0.8660254037844387076, 1.000000000000000000, 0.8660254037844387076, 1.000000000000000000, 0.8660254037844390407, 0.9999999999999996669 ) ) 
 REPRESENTATION_ITEM ( '' )  );
#4332=CARTESIAN_POINT ( 'NONE',  ( -0.7500000000000007772, -14.29903810567666156, -2.666666666666666519 ) ) ;
#4337=CARTESIAN_POINT ( 'NONE',  ( 8.692241771943170539E-17, -11.58044919106553650, -0.7187500006827969301 ) ) ;
#4351=CARTESIAN_POINT ( 'NONE',  ( 1.229367062500000385, -12.29022459553277002, -1.177083334016129967 ) ) ;
#4353=CARTESIAN_POINT ( 'NONE',  ( -1.229367062500000163, -13.00000000000000533, -1.468750000682796486 ) ) ;
#4358=VERTEX_POINT ( 'NONE', #10285 ) ;
#4363=CARTESIAN_POINT ( 'NONE',  ( -0.6146835312500006365, -14.06466310670085562, -0.5104166673494635598 ) ) ;
#4375=CARTESIAN_POINT ( 'NONE',  ( 0.6146835312499993043, -14.06466310670085562, 0.1979166659838698661 ) ) ;
#4378=CIRCLE ( 'NONE', #2189, 4.000000000000000000 ) ;
#4387=CARTESIAN_POINT ( 'NONE',  ( 1.229367062500000163, -13.00000000000000533, -1.343750000682796486 ) ) ;
#4405=CARTESIAN_POINT ( 'NONE',  ( 1.229367062500000163, -13.70977540446723886, -1.760416667349463227 ) ) ;
#4418=CARTESIAN_POINT ( 'NONE',  ( -2.607672531582950546E-16, -14.41955080893447416, 0.03124999931720332663 ) ) ;
#4425=LINE ( 'NONE', #8419, #7622 ) ;
#4439=DIRECTION ( 'NONE',  ( 0.000000000000000000, -0.000000000000000000, 1.000000000000000000 ) ) ;
#4447=CARTESIAN_POINT ( 'NONE',  ( 1.070288219556879694, -11.94905607805280567, 1.518836458664385706E-16 ) ) ;
#4454=CARTESIAN_POINT ( 'NONE',  ( 1.229367062499999719, -13.70977540446724063, -0.7604166673494633377 ) ) ;
#4458=CARTESIAN_POINT ( 'NONE',  ( 1.229367062500000163, -13.70977540446723886, 0.2395833326505366900 ) ) ;
#4471=CARTESIAN_POINT ( 'NONE',  ( 1.500000000000000444, -12.13397459621556607, -2.958333333333333037 ) ) ;
#4508=CARTESIAN_POINT ( 'NONE',  ( -1.229367062500000385, -13.70977540446723886, -0.4270833340161298564 ) ) ;
#4510=CARTESIAN_POINT ( 'NONE',  ( 1.229367062500000163, -12.29022459553277002, -1.177083334016129967 ) ) ;
#4522=CARTESIAN_POINT ( 'NONE',  ( -2.607672531582950546E-16, -14.41955080893447416, -1.968750000682796708 ) ) ;
#4531=ORIENTED_EDGE ( 'NONE', *, *, #748, .T. ) ;
#4538=FACE_OUTER_BOUND ( 'NONE', #2598, .T. ) ;
#4547=DIRECTION ( 'NONE',  ( 1.000000000000000000, 0.000000000000000000, 0.000000000000000000 ) ) ;
#4558=CARTESIAN_POINT ( 'NONE',  ( 1.229367062499999719, -13.70977540446724063, 0.2395833326505366900 ) ) ;
#4571=SURFACE_SIDE_STYLE ('',( #5421 ) ) ;
#4574=CARTESIAN_POINT ( 'NONE',  ( 0.6146835312500001924, -11.93533689329915326, -1.760416667349463449 ) ) ;
#4581=DIRECTION ( 'NONE',  ( 0.8660254037844397068, 0.000000000000000000, -0.4999999999999983347 ) ) ;
#4587=CARTESIAN_POINT ( 'NONE',  ( 1.500000000000000222, -13.00000000000000533, -1.500000000000000000 ) ) ;
#4593=ORIENTED_EDGE ( 'NONE', *, *, #7981, .F. ) ;
#4604=CARTESIAN_POINT ( 'NONE',  ( -3.181725716174720991E-16, -14.73205080756888563, -0.1250000000000001110 ) ) ;
#4610=CARTESIAN_POINT ( 'NONE',  ( 8.692241771943169307E-17, -11.58044919106553294, -2.218750000682796486 ) ) ;
#4620=CARTESIAN_POINT ( 'NONE',  ( 1.500000000000000222, -13.00000000000000533, -3.000000000000000000 ) ) ;
#4621=EDGE_LOOP ( 'NONE', ( #7059, #1773, #6177, #9877 ) ) ;
#4625=CARTESIAN_POINT ( 'NONE',  ( 1.500000000000000222, -13.00000000000000533, 0.000000000000000000 ) ) ;
#4637=STYLED_ITEM ( 'NONE', ( #8940 ), #8917 ) ;
#4657=CARTESIAN_POINT ( 'NONE',  ( 0.000000000000000000, -13.00000000000000533, -3.000000000000000000 ) ) ;
#4662=CARTESIAN_POINT ( 'NONE',  ( 1.229367062500000385, -12.29022459553277002, -2.802083334016129523 ) ) ;
#4670=CARTESIAN_POINT ( 'NONE',  ( -0.7500000000000007772, -14.29903810567666156, -0.6666666666666669627 ) ) ;
#4672=CARTESIAN_POINT ( 'NONE',  ( 1.500000000000000222, -13.00000000000000533, -0.5000000000000000000 ) ) ;
#4680=CARTESIAN_POINT ( 'NONE',  ( 1.500000000000000222, -13.00000000000000533, -0.5000000000000000000 ) ) ;
#4695=LINE ( 'NONE', #2433, #7960 ) ;
#4701=CARTESIAN_POINT ( 'NONE',  ( 0.7499999999999991118, -14.29903810567666333, -1.645833334698926675 ) ) ;
#4707=CYLINDRICAL_SURFACE ( 'NONE', #8467, 1.500000000000000222 ) ;
#4714=CARTESIAN_POINT ( 'NONE',  ( 1.229367062499999719, -13.70977540446724063, -1.385416667349463671 ) ) ;
#4722=DIRECTION ( 'NONE',  ( -0.000000000000000000, -0.000000000000000000, -1.000000000000000000 ) ) ;
#4724=AXIS2_PLACEMENT_3D ( 'NONE', #8173, #1752, #4131 ) ;
#4729=AXIS2_PLACEMENT_3D ( 'NONE', #8629, #1312, #7835 ) ;
#4734=CARTESIAN_POINT ( 'NONE',  ( -3.181725716174720498E-16, -14.73205080756888385, -0.6250000000000001110 ) ) ;
#4738=( BOUNDED_CURVE ( )  B_SPLINE_CURVE ( 2, ( #3309, #4301, #3465, #1824, #879, #4251, #1668, #6689, #4893, #8350, #5103, #9945, #1079, #7547, #3514, #7338, #1231, #3615, #6149, #3769, #10099, #5151, #1131, #4405, #389, #2873, #6999, #489, #10251, #8401, #4353, #1330, #5359, #1983, #5203, #5938, #7593, #4510, #6950, #6793, #9292, #543, #2032, #6842, #6099, #9349, #7755, #9244, #9191, #3717, #8449, #10204, #3565, #1930, #1178, #6039, #8500, #336, #5261, #9401, #1284, #2138, #7811, #10049, #2773, #2825, #2083, #5310, #5986, #7651, #8599, #4458, #2930 ),
 .UNSPECIFIED., .F., .F. ) 
 B_SPLINE_CURVE_WITH_KNOTS ( ( 3, 2, 2, 2, 2, 2, 2, 2, 2, 2, 2, 2, 2, 2, 2, 2, 2, 2, 2, 2, 2, 2, 2, 2, 2, 2, 2, 2, 2, 2, 2, 2, 2, 2, 2, 2, 3 ),
 ( 0.000000000000000000, 0.02777777777777777624, 0.05555555555555555247, 0.08333333333333332871, 0.1111111111111111049, 0.1388888888888888951, 0.1666666666666666574, 0.1944444444444444475, 0.2222222222222222099, 0.2500000000000000000, 0.2777777777777777901, 0.3055555555555555802, 0.3333333333333333148, 0.3611111111111111049, 0.3888888888888888951, 0.4166666666666666852, 0.4444444444444444198, 0.4722222222222222099, 0.5000000000000000000, 0.5277777777777777901, 0.5555555555555555802, 0.5833333333333333703, 0.6111111111111111605, 0.6388888888888888395, 0.6666666666666666297, 0.6944444444444444198, 0.7222222222222222099, 0.7500000000000000000, 0.7777777777777777901, 0.8055555555555555802, 0.8333333333333333703, 0.8611111111111111605, 0.8888888888888888395, 0.9166666666666666297, 0.9444444444444444198, 0.9722222222222222099, 1.000000000000000000 ),
 .UNSPECIFIED. ) 
 CURVE ( )  GEOMETRIC_REPRESENTATION_ITEM ( )  RATIONAL_B_SPLINE_CURVE ( ( 1.000000000000000000, 0.8660254037844387076, 1.000000000000000000, 0.8660254037844387076, 1.000000000000000000, 0.8660254037844387076, 1.000000000000000000, 0.8660254037844387076, 1.000000000000000000, 0.8660254037844387076, 1.000000000000000000, 0.8660254037844387076, 1.000000000000000000, 0.8660254037844387076, 1.000000000000000000, 0.8660254037844387076, 1.000000000000000000, 0.8660254037844387076, 1.000000000000000000, 0.8660254037844387076, 1.000000000000000000, 0.8660254037844387076, 1.000000000000000000, 0.8660254037844387076, 1.000000000000000000, 0.8660254037844387076, 1.000000000000000000, 0.8660254037844387076, 1.000000000000000000, 0.8660254037844387076, 1.000000000000000000, 0.8660254037844387076, 1.000000000000000000, 0.8660254037844387076, 1.000000000000000000, 0.8660254037844387076, 1.000000000000000000, 0.8660254037844387076, 1.000000000000000000, 0.8660254037844387076, 1.000000000000000000, 0.8660254037844387076, 1.000000000000000000, 0.8660254037844387076, 1.000000000000000000, 0.8660254037844387076, 1.000000000000000000, 0.8660254037844387076, 1.000000000000000000, 0.8660254037844387076, 1.000000000000000000, 0.8660254037844387076, 1.000000000000000000, 0.8660254037844387076, 1.000000000000000000, 0.8660254037844387076, 1.000000000000000000, 0.8660254037844387076, 1.000000000000000000, 0.8660254037844387076, 1.000000000000000000, 0.8660254037844387076, 1.000000000000000000, 0.8660254037844387076, 1.000000000000000000, 0.8660254037844387076, 1.000000000000000000, 0.8660254037844387076, 1.000000000000000000, 0.8660254037844387076, 1.000000000000000000, 0.8660254037844387076, 1.000000000000000000 ) ) 
 REPRESENTATION_ITEM ( '' )  );
#4739=ORIENTED_EDGE ( 'NONE', *, *, #8678, .F. ) ;
#4765=CARTESIAN_POINT ( 'NONE',  ( 1.229367062499999719, -13.70977540446724063, -2.260416667349463005 ) ) ;
#4775=MANIFOLD_SOLID_BREP ( 'Thread1', #7956 ) ;
#4789=CARTESIAN_POINT ( 'NONE',  ( 0.000000000000000000, -13.00000000000000533, 2.000000000000000000 ) ) ;
#4794=CARTESIAN_POINT ( 'NONE',  ( 0.7499999999999991118, -14.29903810567666333, -1.083333333333333481 ) ) ;
#4797=DIRECTION ( 'NONE',  ( 0.000000000000000000, 0.000000000000000000, 1.000000000000000000 ) ) ;
#4801=DIRECTION ( 'NONE',  ( 0.000000000000000000, 0.000000000000000000, 1.000000000000000000 ) ) ;
#4808=LINE ( 'NONE', #47, #3216 ) ;
#4817=CARTESIAN_POINT ( 'NONE',  ( -0.7499999999999997780, -11.70096189432334555, 0.1041666653010730748 ) ) ;
#4827=VERTEX_POINT ( 'NONE', #6264 ) ;
#4828=CARTESIAN_POINT ( 'NONE',  ( -2.607672531582950546E-16, -14.41955080893447416, 0.03124999931720332663 ) ) ;
#4836=CARTESIAN_POINT ( 'NONE',  ( 1.070288219556879694, -11.94905607805280567, 1.518836458664385706E-16 ) ) ;
#4844=UNCERTAINTY_MEASURE_WITH_UNIT (LENGTH_MEASURE( 1.000000000000000082E-05 ), #7026, 'distance_accuracy_value', 'NONE');
#4845=CARTESIAN_POINT ( 'NONE',  ( -3.181725716174720498E-16, -14.73205080756888385, -0.1250000000000001110 ) ) ;
#4855=ORIENTED_EDGE ( 'NONE', *, *, #5996, .T. ) ;
#4856=SHAPE_REPRESENTATION_RELATIONSHIP ( 'NONE' , 'NONE' ,  #9732, #8917 ) ;
#4859=DIRECTION ( 'NONE',  ( 0.000000000000000000, 0.000000000000000000, 1.000000000000000000 ) ) ;
#4860=CARTESIAN_POINT ( 'NONE',  ( 1.500000000000000222, -13.00000000000000533, -2.000000000000000000 ) ) ;
#4866=CARTESIAN_POINT ( 'NONE',  ( -0.7499999999999997780, -11.70096189432334555, -0.8958333346989268975 ) ) ;
#4879=CARTESIAN_POINT ( 'NONE',  ( 1.229367062499999719, -13.70977540446724063, -0.3854166673494633932 ) ) ;
#4893=CARTESIAN_POINT ( 'NONE',  ( -0.6146835312500006365, -14.06466310670085562, -2.385416667349463005 ) ) ;
#4912=CARTESIAN_POINT ( 'NONE',  ( -4.000000000000000000, -13.00000000000000533, 2.000000000000000000 ) ) ;
#4921=CARTESIAN_POINT ( 'NONE',  ( 1.500000000000000444, -12.13397459621556607, -1.520833334698926897 ) ) ;
#4923=APPLICATION_CONTEXT ( 'automotive_design' ) ;
#4932=PLANE ( 'NONE',  #4724 ) ;
#4937=CARTESIAN_POINT ( 'NONE',  ( 1.229367062500000385, -12.29022459553277002, -0.3020833340161301339 ) ) ;
#4942=CYLINDRICAL_SURFACE ( 'NONE', #1453, 1.500000000000000222 ) ;
#4966=CARTESIAN_POINT ( 'NONE',  ( 0.7500000000000003331, -11.70096189432334732, -0.4166666666666667407 ) ) ;
#4972=CARTESIAN_POINT ( 'NONE',  ( -0.6146835312500006365, -14.06466310670085562, -0.3854166673494634487 ) ) ;
#4982=CARTESIAN_POINT ( 'NONE',  ( -1.229367062500000163, -13.70977540446723708, -2.052083334016129967 ) ) ;
#5006=EDGE_CURVE ( 'NONE', #6611, #6335, #9361, .T. ) ;
#5018=SURFACE_STYLE_FILL_AREA ( #7244 ) ;
#5027=CARTESIAN_POINT ( 'NONE',  ( 0.6146835312500001924, -11.93533689329915326, -0.6354166673494632267 ) ) ;
#5034=CARTESIAN_POINT ( 'NONE',  ( 1.229367062500000163, -13.70977540446723886, -1.385416667349463449 ) ) ;
#5046=ADVANCED_FACE ( 'NONE', ( #9608 ), #8592, .T. ) ;
#5048=CARTESIAN_POINT ( 'NONE',  ( 0.000000000000000000, -13.00000000000000533, 2.000000000000000000 ) ) ;
#5061=CARTESIAN_POINT ( 'NONE',  ( 0.6146835312499993043, -14.06466310670085562, -2.427083334016129967 ) ) ;
#5062=VERTEX_POINT ( 'NONE', #8748 ) ;
#5073=CARTESIAN_POINT ( 'NONE',  ( -1.229367062500000385, -13.70977540446723886, -1.427083334016129745 ) ) ;
#5083=CARTESIAN_POINT ( 'NONE',  ( 1.229367062500000163, -12.29022459553277002, -0.8020833340161301894 ) ) ;
#5103=CARTESIAN_POINT ( 'NONE',  ( 0.6146835312499993043, -14.06466310670085562, -2.302083334016129967 ) ) ;
#5124=CARTESIAN_POINT ( 'NONE',  ( 0.6146835312500001924, -11.93533689329915326, -2.135416667349463449 ) ) ;
#5127=ORIENTED_EDGE ( 'NONE', *, *, #2607, .F. ) ;
#5136=CARTESIAN_POINT ( 'NONE',  ( 1.229367062500000163, -13.70977540446723886, -0.3854166673494634487 ) ) ;
#5149=CARTESIAN_POINT ( 'NONE',  ( 1.229367062499999719, -13.70977540446724063, -1.260416667349463449 ) ) ;
#5151=CARTESIAN_POINT ( 'NONE',  ( -2.607672531582950546E-16, -14.41955080893447416, -1.843750000682796708 ) ) ;
#5164=CARTESIAN_POINT ( 'NONE',  ( -1.500000000000002220, -13.86602540378444282, -1.270833334698927120 ) ) ;
#5177=CARTESIAN_POINT ( 'NONE',  ( 1.229367062500000385, -12.29022459553277002, -1.177083334016129967 ) ) ;
#5187=CARTESIAN_POINT ( 'NONE',  ( -1.229367062500000163, -13.70977540446723708, -0.05208333401612994656 ) ) ;
#5195=CARTESIAN_POINT ( 'NONE',  ( 1.060575238724907038E-16, -11.26794919243112680, -2.875000000000000000 ) ) ;
#5198=LINE ( 'NONE', #1074, #6589 ) ;
#5200=CARTESIAN_POINT ( 'NONE',  ( -1.229367062500000163, -12.29022459553277002, -2.510416667349463449 ) ) ;
#5203=CARTESIAN_POINT ( 'NONE',  ( 0.6146835312499993043, -14.06466310670085562, -1.302083334016129967 ) ) ;
#5212=CARTESIAN_POINT ( 'NONE',  ( 0.6146835312499993043, -14.06466310670085562, -0.4270833340161298564 ) ) ;
#5222=EDGE_CURVE ( 'NONE', #5062, #4078, #5754, .T. ) ;
#5240=CYLINDRICAL_SURFACE ( 'NONE', #1510, 1.500000000000000222 ) ;
#5245=MECHANICAL_DESIGN_GEOMETRIC_PRESENTATION_REPRESENTATION('',(#8470),#5751);
#5257=CARTESIAN_POINT ( 'NONE',  ( -0.6146835312500006365, -14.06466310670085562, -2.385416667349463005 ) ) ;
#5261=CARTESIAN_POINT ( 'NONE',  ( 0.6146835312499993043, -14.06466310670085562, -0.3020833340161297453 ) ) ;
#5270=EDGE_LOOP ( 'NONE', ( #4324, #7506, #8058, #5535, #6570 ) ) ;
#5273=CARTESIAN_POINT ( 'NONE',  ( -1.229367062500000163, -13.00000000000000533, -1.593750000682796708 ) ) ;
#5278=LINE ( 'NONE', #9309, #9327 ) ;
#5292=FACE_OUTER_BOUND ( 'NONE', #6595, .T. ) ;
#5293=CARTESIAN_POINT ( 'NONE',  ( 1.229367062500000163, -13.00000000000000533, 0.1562499993172034307 ) ) ;
#5307=CARTESIAN_POINT ( 'NONE',  ( 1.229367062499999719, -13.70977540446724063, -0.2604166673494632822 ) ) ;
#5310=CARTESIAN_POINT ( 'NONE',  ( -1.229367062500000163, -13.70977540446723708, 0.07291666598387017140 ) ) ;
#5321=CARTESIAN_POINT ( 'NONE',  ( 0.6146835312499993043, -14.06466310670085562, -1.927083334016129967 ) ) ;
#5339=FACE_OUTER_BOUND ( 'NONE', #6445, .T. ) ;
#5348=CARTESIAN_POINT ( 'NONE',  ( 1.229367062500000163, -13.00000000000000533, -2.843750000682796486 ) ) ;
#5349=CARTESIAN_POINT ( 'NONE',  ( 0.7500000000000003331, -11.70096189432334732, -2.916666666666666963 ) ) ;
#5353=LINE ( 'NONE', #2132, #9617 ) ;
#5356=CARTESIAN_POINT ( 'NONE',  ( -0.6146835312500006365, -14.06466310670085562, -1.510416667349463227 ) ) ;
#5359=CARTESIAN_POINT ( 'NONE',  ( -0.6146835312500006365, -14.06466310670085562, -1.385416667349463227 ) ) ;
#5361=CARTESIAN_POINT ( 'NONE',  ( -0.7500000000000007772, -14.29903810567666156, -2.229166668032259935 ) ) ;
#5370=CARTESIAN_POINT ( 'NONE',  ( -1.229367062500000385, -13.70977540446723886, -0.05208333401612993269 ) ) ;
#5371=ORIENTED_EDGE ( 'NONE', *, *, #1152, .T. ) ;
#5382=ORIENTED_EDGE ( 'NONE', *, *, #6829, .T. ) ;
#5401=EDGE_CURVE ( 'NONE', #8892, #9635, #6775, .T. ) ;
#5402=CARTESIAN_POINT ( 'NONE',  ( -3.181725716174720991E-16, -14.73205080756888563, -1.125000000000000222 ) ) ;
#5407=CARTESIAN_POINT ( 'NONE',  ( -0.6146835312499998594, -11.93533689329915326, -2.677083334016129967 ) ) ;
#5419=CARTESIAN_POINT ( 'NONE',  ( 0.7499999999999991118, -14.29903810567666333, -0.1458333346989267310 ) ) ;
#5421=SURFACE_STYLE_FILL_AREA ( #3095 ) ;
#5425=CARTESIAN_POINT ( 'NONE',  ( 0.6146835312499993043, -14.06466310670085562, -1.427083334016129967 ) ) ;
#5433=CARTESIAN_POINT ( 'NONE',  ( -1.500000000000000222, -13.00000000000000533, -2.312500001365593860 ) ) ;
#5439=ORIENTED_EDGE ( 'NONE', *, *, #5557, .F. ) ;
#5451=DIRECTION ( 'NONE',  ( 0.000000000000000000, 0.000000000000000000, -1.000000000000000000 ) ) ;
#5455=CARTESIAN_POINT ( 'NONE',  ( 1.060575238724907038E-16, -11.26794919243112680, -2.375000000000000444 ) ) ;
#5457=CARTESIAN_POINT ( 'NONE',  ( -0.7500000000000007772, -14.29903810567666156, -1.166666666666666741 ) ) ;
#5460=CARTESIAN_POINT ( 'NONE',  ( 1.229367062500000385, -12.29022459553277002, -0.1770833340161300229 ) ) ;
#5466=CARTESIAN_POINT ( 'NONE',  ( 1.499999999999999778, -13.86602540378444637, -2.104166668032260379 ) ) ;
#5470=CARTESIAN_POINT ( 'NONE',  ( -1.500000000000002220, -13.86602540378444282, -1.708333333333333481 ) ) ;
#5476=CARTESIAN_POINT ( 'NONE',  ( -3.181725716174720498E-16, -14.73205080756888385, -2.125000000000000000 ) ) ;
#5477=EDGE_LOOP ( 'NONE', ( #4051, #650, #5371, #989 ) ) ;
#5481=CARTESIAN_POINT ( 'NONE',  ( 1.060575238724907038E-16, -11.26794919243112680, -0.8750000000000003331 ) ) ;
#5488=MECHANICAL_DESIGN_GEOMETRIC_PRESENTATION_REPRESENTATION('',(#4637),#927);
#5491=CIRCLE ( 'NONE', #3981, 1.500000000000000222 ) ;
#5492=CARTESIAN_POINT ( 'NONE',  ( 1.500000000000000222, -13.00000000000000533, -1.562500001365593416 ) ) ;
#5501=CARTESIAN_POINT ( 'NONE',  ( 0.7499999999999991118, -14.29903810567666333, 0.3541666653010728805 ) ) ;
#5504=ORIENTED_EDGE ( 'NONE', *, *, #2486, .F. ) ;
#5505=CARTESIAN_POINT ( 'NONE',  ( -3.181725716174720991E-16, -14.73205080756888563, -0.6875000013655935271 ) ) ;
#5515=CARTESIAN_POINT ( 'NONE',  ( 0.6146835312499993043, -14.06466310670085562, -1.427083334016129967 ) ) ;
#5531=CARTESIAN_POINT ( 'NONE',  ( 1.500000000000000444, -12.13397459621556607, -0.9583333333333337034 ) ) ;
#5534=CARTESIAN_POINT ( 'NONE',  ( -0.7499999999999997780, -11.70096189432334555, -0.8333333333333334814 ) ) ;
#5535=ORIENTED_EDGE ( 'NONE', *, *, #215, .T. ) ;
#5552=CARTESIAN_POINT ( 'NONE',  ( -2.607672531582950546E-16, -14.41955080893447416, -2.343750000682796930 ) ) ;
#5553=ADVANCED_FACE ( 'NONE', ( #8641 ), #6139, .T. ) ;
#5557=EDGE_CURVE ( 'NONE', #7636, #9635, #7248, .T. ) ;
#5580=CARTESIAN_POINT ( 'NONE',  ( 0.7499999999999991118, -14.29903810567666333, -1.583333333333333481 ) ) ;
#5585=CARTESIAN_POINT ( 'NONE',  ( 1.500000000000000222, -13.00000000000000533, -1.000000000000000000 ) ) ;
#5598=EDGE_CURVE ( 'NONE', #8600, #8355, #9023, .T. ) ;
#5603=CARTESIAN_POINT ( 'NONE',  ( 1.060575238724907038E-16, -11.26794919243112680, -1.875000000000000222 ) ) ;
#5609=CARTESIAN_POINT ( 'NONE',  ( -0.7500000000000007772, -14.29903810567666156, -0.2291666680322604066 ) ) ;
#5610=DIRECTION ( 'NONE',  ( 0.000000000000000000, 0.000000000000000000, 1.000000000000000000 ) ) ;
#5619=CARTESIAN_POINT ( 'NONE',  ( 0.6146835312500001924, -11.93533689329915326, -0.2604166673494633377 ) ) ;
#5629=DIRECTION ( 'NONE',  ( 0.000000000000000000, 0.000000000000000000, 1.000000000000000000 ) ) ;
#5634=CARTESIAN_POINT ( 'NONE',  ( -0.7500000000000007772, -14.29903810567666156, -0.1666666666666669627 ) ) ;
#5640=ORIENTED_EDGE ( 'NONE', *, *, #7781, .F. ) ;
#5659=CARTESIAN_POINT ( 'NONE',  ( -1.500000000000000000, -12.13397459621556607, 0.1458333319677399265 ) ) ;
#5679=AXIS2_PLACEMENT_3D ( 'NONE', #1560, #4722, #7381 ) ;
#5681=CARTESIAN_POINT ( 'NONE',  ( 1.500000000000000222, -13.00000000000000533, -2.500000000000000000 ) ) ;
#5683=CARTESIAN_POINT ( 'NONE',  ( 0.7499999999999991118, -14.29903810567666333, -0.08333333333333370341 ) ) ;
#5695=EDGE_CURVE ( 'NONE', #4827, #1061, #6441, .T. ) ;
#5704=CARTESIAN_POINT ( 'NONE',  ( -1.500000000000000000, -12.13397459621556607, -0.3541666680322600458 ) ) ;
#5722=DIRECTION ( 'NONE',  ( 1.000000000000000000, 0.000000000000000000, 0.000000000000000000 ) ) ;
#5725=FACE_OUTER_BOUND ( 'NONE', #6587, .T. ) ;
#5732=ADVANCED_FACE ( 'NONE', ( #3977 ), #9500, .T. ) ;
#5751=( GEOMETRIC_REPRESENTATION_CONTEXT ( 3 ) GLOBAL_UNCERTAINTY_ASSIGNED_CONTEXT ( ( #7677 ) ) GLOBAL_UNIT_ASSIGNED_CONTEXT ( ( #8562, #6904, #10158 ) ) REPRESENTATION_CONTEXT ( 'NONE', 'WORKASPACE' ) );
#5754=( BOUNDED_CURVE ( )  B_SPLINE_CURVE ( 2, ( #7860, #2244, #5361, #9405, #9515, #5466, #6205 ),
 .UNSPECIFIED., .F., .F. ) 
 B_SPLINE_CURVE_WITH_KNOTS ( ( 3, 2, 2, 3 ),
 ( 0.08333333333333325932, 0.1111111111111110494, 0.1388888888888888673, 0.1666666666666666574 ),
 .UNSPECIFIED. ) 
 CURVE ( )  GEOMETRIC_REPRESENTATION_ITEM ( )  RATIONAL_B_SPLINE_CURVE ( ( 1.000000000000000222, 0.8660254037844383745, 1.000000000000000000, 0.8660254037844387076, 1.000000000000000000, 0.8660254037844387076, 1.000000000000000000 ) ) 
 REPRESENTATION_ITEM ( '' )  );
#5759=VECTOR ( 'NONE', #10260, 1000.000000000000000 ) ;
#5760=CARTESIAN_POINT ( 'NONE',  ( 1.229367062500000385, -12.29022459553277002, -0.6770833340161300784 ) ) ;
#5762=ORIENTED_EDGE ( 'NONE', *, *, #8502, .F. ) ;
#5768=CARTESIAN_POINT ( 'NONE',  ( -1.229367062500000163, -12.29022459553277002, -1.635416667349463227 ) ) ;
#5771=CARTESIAN_POINT ( 'NONE',  ( -0.6146835312499998594, -11.93533689329915326, -0.1770833340161300506 ) ) ;
#5803=CARTESIAN_POINT ( 'NONE',  ( -1.499999999999999778, -12.13397459621556784, -0.2916666666666666852 ) ) ;
#5809=CARTESIAN_POINT ( 'NONE',  ( 0.6146835312500001924, -11.93533689329915326, -1.135416667349463227 ) ) ;
#5810=VECTOR ( 'NONE', #5451, 1000.000000000000000 ) ;
#5813=( BOUNDED_CURVE ( )  B_SPLINE_CURVE ( 2, ( #1106, #9115, #4332, #3285, #6510, #517, #2009 ),
 .UNSPECIFIED., .F., .F. ) 
 B_SPLINE_CURVE_WITH_KNOTS ( ( 3, 2, 2, 3 ),
 ( 0.08333333333333339810, 0.1111111111111111466, 0.1388888888888889228, 0.1666666666666666574 ),
 .UNSPECIFIED. ) 
 CURVE ( )  GEOMETRIC_REPRESENTATION_ITEM ( )  RATIONAL_B_SPLINE_CURVE ( ( 0.9999999999999996669, 0.8660254037844390407, 1.000000000000000000, 0.8660254037844387076, 1.000000000000000000, 0.8660254037844387076, 1.000000000000000000 ) ) 
 REPRESENTATION_ITEM ( '' )  );
#5815=CYLINDRICAL_SURFACE ( 'NONE', #1030, 1.500000000000000222 ) ;
#5821=CARTESIAN_POINT ( 'NONE',  ( -0.6146835312500006365, -14.06466310670085562, -1.510416667349463227 ) ) ;
#5861=CARTESIAN_POINT ( 'NONE',  ( -0.6146835312499998594, -11.93533689329915326, -0.05208333401612993963 ) ) ;
#5863=VERTEX_POINT ( 'NONE', #2495 ) ;
#5865=DIRECTION ( 'NONE',  ( -0.8660254037844402619, 0.000000000000000000, -0.4999999999999972244 ) ) ;
#5866=CARTESIAN_POINT ( 'NONE',  ( 1.500000000000000222, -12.13397459621556784, -1.020833334698926897 ) ) ;
#5869=CARTESIAN_POINT ( 'NONE',  ( -1.229367062500000163, -13.70977540446723708, -1.552083334016130189 ) ) ;
#5876=EDGE_CURVE ( 'NONE', #10421, #1372, #9766, .T. ) ;
#5882=CARTESIAN_POINT ( 'NONE',  ( 0.6146835312499993043, -14.06466310670085562, -1.802083334016129745 ) ) ;
#5898=EDGE_CURVE ( 'NONE', #8600, #9521, #5491, .T. ) ;
#5901=AXIS2_PLACEMENT_3D ( 'NONE', #4789, #4147, #7228 ) ;
#5903=DIRECTION ( 'NONE',  ( 1.000000000000000000, 0.000000000000000000, 0.000000000000000000 ) ) ;
#5911=CARTESIAN_POINT ( 'NONE',  ( -0.6146835312500006365, -14.06466310670085562, -1.885416667349463227 ) ) ;
#5920=CARTESIAN_POINT ( 'NONE',  ( -0.6146835312499998594, -11.93533689329915326, -1.677083334016129967 ) ) ;
#5924=CARTESIAN_POINT ( 'NONE',  ( 0.000000000000000000, -13.00000000000000533, 0.000000000000000000 ) ) ;
#5936=CARTESIAN_POINT ( 'NONE',  ( 1.229367062500000163, -13.00000000000000533, -1.218750000682796486 ) ) ;
#5938=CARTESIAN_POINT ( 'NONE',  ( 1.229367062500000163, -13.70977540446723886, -1.260416667349463449 ) ) ;
#5947=CARTESIAN_POINT ( 'NONE',  ( -1.229367062500000163, -12.29022459553277002, -2.135416667349463449 ) ) ;
#5948=ORIENTED_EDGE ( 'NONE', *, *, #8031, .T. ) ;
#5960=CARTESIAN_POINT ( 'NONE',  ( 0.6146835312499993043, -14.06466310670085562, -0.8020833340161299674 ) ) ;
#5971=CARTESIAN_POINT ( 'NONE',  ( -0.6146835312499998594, -11.93533689329915326, -0.1770833340161300506 ) ) ;
#5981=CARTESIAN_POINT ( 'NONE',  ( -1.500000000000000222, -13.00000000000000533, -0.7500000000000002220 ) ) ;
#5983=CARTESIAN_POINT ( 'NONE',  ( 1.229367062500000385, -12.29022459553277002, -2.677083334016129967 ) ) ;
#5986=CARTESIAN_POINT ( 'NONE',  ( -0.6146835312500006365, -14.06466310670085562, 0.1145833326505365929 ) ) ;
#5994=VECTOR ( 'NONE', #4216, 1000.000000000000000 ) ;
#5996=EDGE_CURVE ( 'NONE', #8355, #6611, #5813, .T. ) ;
#5999=CARTESIAN_POINT ( 'NONE',  ( 1.229367062500000385, -12.29022459553277002, -0.8020833340161301894 ) ) ;
#6005=CARTESIAN_POINT ( 'NONE',  ( 1.500000000000000222, -13.00000000000000533, -0.5000000000000000000 ) ) ;
#6031=CARTESIAN_POINT ( 'NONE',  ( -0.7499999999999997780, -11.70096189432334555, -2.833333333333333481 ) ) ;
#6036=CARTESIAN_POINT ( 'NONE',  ( 8.692241771943169307E-17, -11.58044919106553294, -1.093750000682796486 ) ) ;
#6039=CARTESIAN_POINT ( 'NONE',  ( -1.229367062500000163, -13.70977540446723708, -0.4270833340161298564 ) ) ;
#6044=LINE ( 'NONE', #8407, #3062 ) ;
#6049=CARTESIAN_POINT ( 'NONE',  ( 1.229367062500000163, -13.00000000000000533, -1.343750000682796486 ) ) ;
#6080=VECTOR ( 'NONE', #9973, 1000.000000000000000 ) ;
#6095=CARTESIAN_POINT ( 'NONE',  ( 1.229367062500000163, -13.00000000000000533, -0.7187500006827964860 ) ) ;
#6099=CARTESIAN_POINT ( 'NONE',  ( -0.6146835312500006365, -14.06466310670085562, -0.8854166673494632267 ) ) ;
#6111=CARTESIAN_POINT ( 'NONE',  ( -1.500000000000000222, -13.00000000000000533, -2.750000000000000000 ) ) ;
#6137=CARTESIAN_POINT ( 'NONE',  ( 1.500000000000000222, -13.00000000000000533, -0.5625000013655934161 ) ) ;
#6139=CYLINDRICAL_SURFACE ( 'NONE', #428, 1.500000000000000222 ) ;
#6147=CARTESIAN_POINT ( 'NONE',  ( 0.6146835312500001924, -11.93533689329915326, -2.260416667349463449 ) ) ;
#6149=CARTESIAN_POINT ( 'NONE',  ( -1.229367062500000163, -13.00000000000000533, -1.968750000682796708 ) ) ;
#6154=( BOUNDED_CURVE ( )  B_SPLINE_CURVE ( 2, ( #3176, #5164, #6648, #3370, #4166, #938, #987 ),
 .UNSPECIFIED., .F., .T. ) 
 B_SPLINE_CURVE_WITH_KNOTS ( ( 3, 2, 2, 3 ),
 ( 0.4166666666666666297, 0.4444444444444443643, 0.4722222222222222099, 0.5000000000000000000 ),
 .UNSPECIFIED. ) 
 CURVE ( )  GEOMETRIC_REPRESENTATION_ITEM ( )  RATIONAL_B_SPLINE_CURVE ( ( 1.000000000000000222, 0.8660254037844384856, 1.000000000000000000, 0.8660254037844387076, 1.000000000000000000, 0.8660254037844387076, 1.000000000000000000 ) ) 
 REPRESENTATION_ITEM ( '' )  );
#6162=CARTESIAN_POINT ( 'NONE',  ( -1.229367062500000385, -13.70977540446723886, -0.5520833340161299674 ) ) ;
#6177=ORIENTED_EDGE ( 'NONE', *, *, #7866, .F. ) ;
#6191=CARTESIAN_POINT ( 'NONE',  ( -1.500000000000000222, -13.00000000000000533, -3.000000000000000000 ) ) ;
#6194=DIRECTION ( 'NONE',  ( 1.000000000000000000, 0.000000000000000000, 0.000000000000000000 ) ) ;
#6197=CARTESIAN_POINT ( 'NONE',  ( -1.500000000000003775, -13.86602540378444104, -1.208333333333333703 ) ) ;
#6200=CARTESIAN_POINT ( 'NONE',  ( 1.229367062500000163, -13.00000000000000533, -2.843750000682796486 ) ) ;
#6204=ORIENTED_EDGE ( 'NONE', *, *, #6377, .F. ) ;
#6205=CARTESIAN_POINT ( 'NONE',  ( 1.500000000000000222, -13.00000000000000533, -2.062500001365593416 ) ) ;
#6213=CARTESIAN_POINT ( 'NONE',  ( 8.692241771943169307E-17, -11.58044919106553294, -1.718750000682796708 ) ) ;
#6217=CARTESIAN_POINT ( 'NONE',  ( 1.060575238724907038E-16, -11.26794919243112680, -2.437500001365593860 ) ) ;
#6218=VERTEX_POINT ( 'NONE', #5492 ) ;
#6225=VERTEX_POINT ( 'NONE', #6285 ) ;
#6227=CARTESIAN_POINT ( 'NONE',  ( -1.500000000000000222, -13.00000000000000533, -1.750000000000000000 ) ) ;
#6235=ORIENTED_EDGE ( 'NONE', *, *, #748, .F. ) ;
#6250=CARTESIAN_POINT ( 'NONE',  ( -1.229367062500000163, -13.00000000000000533, -1.593750000682796708 ) ) ;
#6255=VERTEX_POINT ( 'NONE', #6227 ) ;
#6264=CARTESIAN_POINT ( 'NONE',  ( -1.500000000000000222, -13.00000000000000533, -0.8125000013655935271 ) ) ;
#6267=CARTESIAN_POINT ( 'NONE',  ( 0.7499999999999991118, -14.29903810567666333, -2.583333333333333481 ) ) ;
#6278=CARTESIAN_POINT ( 'NONE',  ( 1.229367062500000163, -13.70977540446723886, 0.1145833326505366068 ) ) ;
#6285=CARTESIAN_POINT ( 'NONE',  ( 1.500000000000000222, -13.00000000000000533, -0.06250000136559345776 ) ) ;
#6292=CARTESIAN_POINT ( 'NONE',  ( -1.500000000000000666, -13.86602540378444459, -1.770833334698926897 ) ) ;
#6303=CARTESIAN_POINT ( 'NONE',  ( 1.229367062499999719, -13.70977540446724063, -1.885416667349463449 ) ) ;
#6307=AXIS2_PLACEMENT_3D ( 'NONE', #2612, #7487, #228 ) ;
#6314=CARTESIAN_POINT ( 'NONE',  ( 1.500000000000000222, -13.00000000000000533, -0.5625000013655934161 ) ) ;
#6319=CARTESIAN_POINT ( 'NONE',  ( 1.500000000000000000, -13.86602540378444459, -1.041666666666666741 ) ) ;
#6322=ORIENTED_EDGE ( 'NONE', *, *, #3507, .F. ) ;
#6335=VERTEX_POINT ( 'NONE', #9705 ) ;
#6349=CARTESIAN_POINT ( 'NONE',  ( -3.181725716174720498E-16, -14.73205080756888385, 0.3124999986344064729 ) ) ;
#6351=EDGE_CURVE ( 'NONE', #252, #7070, #2587, .T. ) ;
#6362=CARTESIAN_POINT ( 'NONE',  ( -1.229367062500000163, -12.29022459553277002, -0.1354166673494631989 ) ) ;
#6377=EDGE_CURVE ( 'NONE', #8600, #8955, #3374, .T. ) ;
#6379=CARTESIAN_POINT ( 'NONE',  ( 0.7499999999999991118, -14.29903810567666333, -2.083333333333333481 ) ) ;
#6380=ORIENTED_EDGE ( 'NONE', *, *, #10438, .F. ) ;
#6393=ORIENTED_EDGE ( 'NONE', *, *, #1152, .F. ) ;
#6399=CARTESIAN_POINT ( 'NONE',  ( -1.500000000000000666, -13.86602540378444459, -1.270833334698926897 ) ) ;
#6410=CARTESIAN_POINT ( 'NONE',  ( 1.229367062500000163, -13.00000000000000533, -0.8437500006827965970 ) ) ;
#6418=ORIENTED_EDGE ( 'NONE', *, *, #10438, .T. ) ;
#6420=EDGE_CURVE ( 'NONE', #6225, #9635, #7405, .T. ) ;
#6421=CARTESIAN_POINT ( 'NONE',  ( 1.500000000000000222, -13.00000000000000533, -1.500000000000000000 ) ) ;
#6422=DIRECTION ( 'NONE',  ( 1.000000000000000000, 0.000000000000000000, 0.000000000000000000 ) ) ;
#6427=UNCERTAINTY_MEASURE_WITH_UNIT (LENGTH_MEASURE( 1.000000000000000082E-05 ), #1683, 'distance_accuracy_value', 'NONE');
#6429=CARTESIAN_POINT ( 'NONE',  ( -1.500000000000000222, -13.00000000000000533, -0.2500000000000002220 ) ) ;
#6432=EDGE_CURVE ( 'NONE', #9635, #8892, #774, .T. ) ;
#6441=( BOUNDED_CURVE ( )  B_SPLINE_CURVE ( 2, ( #849, #2334, #2282, #5505, #8693, #1544, #7148 ),
 .UNSPECIFIED., .F., .T. ) 
 B_SPLINE_CURVE_WITH_KNOTS ( ( 3, 2, 2, 3 ),
 ( 0.5833333333333332593, 0.6111111111111110494, 0.6388888888888888395, 0.6666666666666666297 ),
 .UNSPECIFIED. ) 
 CURVE ( )  GEOMETRIC_REPRESENTATION_ITEM ( )  RATIONAL_B_SPLINE_CURVE ( ( 1.000000000000000444, 0.8660254037844381525, 1.000000000000000000, 0.8660254037844387076, 1.000000000000000000, 0.8660254037844387076, 1.000000000000000000 ) ) 
 REPRESENTATION_ITEM ( '' )  );
#6445=EDGE_LOOP ( 'NONE', ( #1578, #3059 ) ) ;
#6455=CARTESIAN_POINT ( 'NONE',  ( 0.7499999999999991118, -14.29903810567666333, -1.145833334698926897 ) ) ;
#6469=SHAPE_DEFINITION_REPRESENTATION ( #7058, #9732 ) ;
#6475=FACE_OUTER_BOUND ( 'NONE', #1532, .T. ) ;
#6481=CARTESIAN_POINT ( 'NONE',  ( -1.500000000000000000, -12.13397459621556607, -1.291666666666666963 ) ) ;
#6497=CARTESIAN_POINT ( 'NONE',  ( 1.500000000000000222, -12.13397459621556784, -1.958333333333333925 ) ) ;
#6505=CARTESIAN_POINT ( 'NONE',  ( 0.6146835312500001924, -11.93533689329915326, -2.635416667349463449 ) ) ;
#6510=CARTESIAN_POINT ( 'NONE',  ( 0.7499999999999991118, -14.29903810567666333, -2.583333333333333481 ) ) ;
#6525=AXIS2_PLACEMENT_3D ( 'NONE', #7056, #7004, #7226 ) ;
#6559=CARTESIAN_POINT ( 'NONE',  ( -0.6146835312499998594, -11.93533689329915326, -2.552083334016129967 ) ) ;
#6567=FACE_OUTER_BOUND ( 'NONE', #2841, .T. ) ;
#6568=CARTESIAN_POINT ( 'NONE',  ( 0.6146835312500001924, -11.93533689329915326, -2.260416667349463449 ) ) ;
#6570=ORIENTED_EDGE ( 'NONE', *, *, #5996, .F. ) ;
#6571=CARTESIAN_POINT ( 'NONE',  ( -1.229367062500000385, -13.70977540446723886, -0.05208333401612993269 ) ) ;
#6587=EDGE_LOOP ( 'NONE', ( #6984, #1879, #988, #6908 ) ) ;
#6589=VECTOR ( 'NONE', #8243, 1000.000000000000000 ) ;
#6595=EDGE_LOOP ( 'NONE', ( #6882, #820, #9700, #5640 ) ) ;
#6600=( NAMED_UNIT ( * ) SI_UNIT ( $, .STERADIAN. ) SOLID_ANGLE_UNIT ( ) );
#6603=ORIENTED_EDGE ( 'NONE', *, *, #5598, .F. ) ;
#6611=VERTEX_POINT ( 'NONE', #7721 ) ;
#6613=CARTESIAN_POINT ( 'NONE',  ( 8.692241771943169307E-17, -11.58044919106553294, -2.093750000682796486 ) ) ;
#6619=DIRECTION ( 'NONE',  ( 0.000000000000000000, 0.000000000000000000, 1.000000000000000000 ) ) ;
#6624=CARTESIAN_POINT ( 'NONE',  ( 1.229367062500000163, -12.29022459553277002, -1.302083334016129967 ) ) ;
#6648=CARTESIAN_POINT ( 'NONE',  ( -0.7500000000000007772, -14.29903810567666156, -1.229166668032260157 ) ) ;
#6652=CARTESIAN_POINT ( 'NONE',  ( 0.000000000000000000, -13.00000000000000533, 0.000000000000000000 ) ) ;
#6653=CARTESIAN_POINT ( 'NONE',  ( 1.500000000000000222, -13.00000000000000533, -0.5000000000000000000 ) ) ;
#6659=CARTESIAN_POINT ( 'NONE',  ( -2.607672531582950546E-16, -14.41955080893447416, -0.8437500006827965970 ) ) ;
#6660=EDGE_CURVE ( 'NONE', #274, #2223, #415, .T. ) ;
#6663=ORIENTED_EDGE ( 'NONE', *, *, #7781, .T. ) ;
#6667=ORIENTED_EDGE ( 'NONE', *, *, #1033, .T. ) ;
#6668=AXIS2_PLACEMENT_3D ( 'NONE', #3016, #9274, #4439 ) ;
#6670=CARTESIAN_POINT ( 'NONE',  ( -1.229367062500000163, -12.29022459553277002, -2.135416667349463449 ) ) ;
#6686=CARTESIAN_POINT ( 'NONE',  ( -2.607672531582950546E-16, -14.41955080893447416, -2.343750000682796930 ) ) ;
#6689=CARTESIAN_POINT ( 'NONE',  ( -1.229367062500000163, -13.70977540446723708, -2.427083334016129967 ) ) ;
#6700=CARTESIAN_POINT ( 'NONE',  ( 8.692241771943169307E-17, -11.58044919106553294, -2.218750000682796486 ) ) ;
#6701=ORIENTED_EDGE ( 'NONE', *, *, #2389, .F. ) ;
#6705=DIRECTION ( 'NONE',  ( 1.000000000000000000, 0.000000000000000000, 0.000000000000000000 ) ) ;
#6711=CARTESIAN_POINT ( 'NONE',  ( 0.6146835312500001924, -11.93533689329915326, -1.635416667349463227 ) ) ;
#6716=CARTESIAN_POINT ( 'NONE',  ( -0.6146835312500006365, -14.06466310670085562, -1.010416667349463227 ) ) ;
#6728=CARTESIAN_POINT ( 'NONE',  ( -0.6146835312499998594, -11.93533689329915326, -2.552083334016129967 ) ) ;
#6731=DIRECTION ( 'NONE',  ( 0.000000000000000000, 0.000000000000000000, 1.000000000000000000 ) ) ;
#6738=VECTOR ( 'NONE', #9333, 1000.000000000000000 ) ;
#6751=VERTEX_POINT ( 'NONE', #9728 ) ;
#6761=CARTESIAN_POINT ( 'NONE',  ( 0.6146835312499993043, -14.06466310670085562, -1.302083334016129967 ) ) ;
#6772=CARTESIAN_POINT ( 'NONE',  ( -1.229367062500000163, -13.00000000000000533, -2.593750000682796486 ) ) ;
#6775=CIRCLE ( 'NONE', #7292, 1.500000000000000222 ) ;
#6793=CARTESIAN_POINT ( 'NONE',  ( 8.692241771943170539E-17, -11.58044919106553650, -1.093750000682796486 ) ) ;
#6804=CARTESIAN_POINT ( 'NONE',  ( -1.229367062500000163, -12.29022459553277002, -0.6354166673494632267 ) ) ;
#6816=CARTESIAN_POINT ( 'NONE',  ( -1.229367062500000385, -13.70977540446723886, -1.927083334016129745 ) ) ;
#6829=EDGE_CURVE ( 'NONE', #2259, #6218, #8608, .T. ) ;
#6834=CARTESIAN_POINT ( 'NONE',  ( -0.7500000000000007772, -14.29903810567666156, -0.1666666666666669627 ) ) ;
#6839=( BOUNDED_CURVE ( )  B_SPLINE_CURVE ( 2, ( #1750, #5866, #9071, #113, #7572, #1107, #1805 ),
 .UNSPECIFIED., .F., .F. ) 
 B_SPLINE_CURVE_WITH_KNOTS ( ( 3, 2, 2, 3 ),
 ( 0.5000000000000000000, 0.5277777777777777901, 0.5555555555555554692, 0.5833333333333332593 ),
 .UNSPECIFIED. ) 
 CURVE ( )  GEOMETRIC_REPRESENTATION_ITEM ( )  RATIONAL_B_SPLINE_CURVE ( ( 1.000000000000000000, 0.8660254037844387076, 1.000000000000000000, 0.8660254037844387076, 1.000000000000000000, 0.8660254037844392627, 0.9999999999999994449 ) ) 
 REPRESENTATION_ITEM ( '' )  );
#6840=FACE_OUTER_BOUND ( 'NONE', #2627, .T. ) ;
#6842=CARTESIAN_POINT ( 'NONE',  ( -1.229367062500000163, -13.70977540446723708, -0.9270833340161298564 ) ) ;
#6855=CARTESIAN_POINT ( 'NONE',  ( 8.692241771943169307E-17, -11.58044919106553294, -1.218750000682796930 ) ) ;
#6872=ADVANCED_FACE ( 'NONE', ( #8759 ), #10478, .T. ) ;
#6882=ORIENTED_EDGE ( 'NONE', *, *, #2279, .F. ) ;
#6886=CARTESIAN_POINT ( 'NONE',  ( -3.181725716174720991E-16, -14.73205080756888563, 0.3124999986344064173 ) ) ;
#6893=CARTESIAN_POINT ( 'NONE',  ( -0.6146835312500006365, -14.06466310670085562, -0.3854166673494634487 ) ) ;
#6904=( NAMED_UNIT ( * ) PLANE_ANGLE_UNIT ( ) SI_UNIT ( $, .RADIAN. ) );
#6906=CARTESIAN_POINT ( 'NONE',  ( 8.692241771943169307E-17, -11.58044919106553294, -0.7187500006827969301 ) ) ;
#6908=ORIENTED_EDGE ( 'NONE', *, *, #215, .F. ) ;
#6929=AXIS2_PLACEMENT_3D ( 'NONE', #8378, #10031, #3338 ) ;
#6935=CARTESIAN_POINT ( 'NONE',  ( 0.7500000000000003331, -11.70096189432334732, 0.02083333196773980503 ) ) ;
#6945=CARTESIAN_POINT ( 'NONE',  ( -1.229367062500000163, -12.29022459553277002, -1.635416667349463227 ) ) ;
#6950=CARTESIAN_POINT ( 'NONE',  ( 0.6146835312500001924, -11.93533689329915326, -1.135416667349463227 ) ) ;
#6962=CARTESIAN_POINT ( 'NONE',  ( 0.6146835312499993043, -14.06466310670085562, -0.9270833340161300784 ) ) ;
#6973=ORIENTED_EDGE ( 'NONE', *, *, #7796, .F. ) ;
#6978=CARTESIAN_POINT ( 'NONE',  ( -1.500000000000000222, -13.00000000000000533, -0.2500000000000002220 ) ) ;
#6984=ORIENTED_EDGE ( 'NONE', *, *, #8249, .T. ) ;
#6985=CARTESIAN_POINT ( 'NONE',  ( -1.500000000000000222, -13.00000000000000533, -0.3125000013655936937 ) ) ;
#6996=CARTESIAN_POINT ( 'NONE',  ( 0.6146835312499993043, -14.06466310670085562, -0.3020833340161297453 ) ) ;
#6999=CARTESIAN_POINT ( 'NONE',  ( 0.6146835312500001924, -11.93533689329915326, -1.635416667349463227 ) ) ;
#7004=DIRECTION ( 'NONE',  ( 0.000000000000000000, 0.000000000000000000, 1.000000000000000000 ) ) ;
#7011=CARTESIAN_POINT ( 'NONE',  ( -0.6146835312499998594, -11.93533689329915326, -0.6770833340161300784 ) ) ;
#7026=( LENGTH_UNIT ( ) NAMED_UNIT ( * ) SI_UNIT ( .MILLI., .METRE. ) );
#7048=CARTESIAN_POINT ( 'NONE',  ( 1.229367062500000163, -13.00000000000000533, 0.2812499993172035695 ) ) ;
#7056=CARTESIAN_POINT ( 'NONE',  ( 0.000000000000000000, -13.00000000000000533, -3.000000000000000000 ) ) ;
#7058=PRODUCT_DEFINITION_SHAPE ( 'NONE', 'NONE',  #1276 ) ;
#7059=ORIENTED_EDGE ( 'NONE', *, *, #3507, .T. ) ;
#7064=CARTESIAN_POINT ( 'NONE',  ( -1.500000000000000000, -12.13397459621556607, -0.2916666666666666852 ) ) ;
#7069=CARTESIAN_POINT ( 'NONE',  ( 0.7500000000000003331, -11.70096189432334732, -2.479166668032260379 ) ) ;
#7070=VERTEX_POINT ( 'NONE', #2235 ) ;
#7088=CARTESIAN_POINT ( 'NONE',  ( -1.500000000000000000, -12.13397459621556607, -1.854166668032260157 ) ) ;
#7089=CARTESIAN_POINT ( 'NONE',  ( 0.7500000000000003331, -11.70096189432334732, -0.4791666680322602123 ) ) ;
#7090=CARTESIAN_POINT ( 'NONE',  ( 0.000000000000000000, 0.000000000000000000, 0.000000000000000000 ) ) ;
#7094=CIRCLE ( 'NONE', #5901, 4.000000000000000000 ) ;
#7097=CARTESIAN_POINT ( 'NONE',  ( 1.499999999999999778, -13.86602540378444637, -1.041666666666666963 ) ) ;
#7098=AXIS2_PLACEMENT_3D ( 'NONE', #8480, #1365, #1264 ) ;
#7102=CARTESIAN_POINT ( 'NONE',  ( 1.229367062499999719, -13.70977540446724063, -2.385416667349463005 ) ) ;
#7109=CARTESIAN_POINT ( 'NONE',  ( -1.500000000000000666, -13.86602540378444637, -0.7083333333333333703 ) ) ;
#7120=CARTESIAN_POINT ( 'NONE',  ( 1.500000000000000000, -13.86602540378444459, -1.541666666666666963 ) ) ;
#7121=ORIENTED_EDGE ( 'NONE', *, *, #859, .T. ) ;
#7143=CARTESIAN_POINT ( 'NONE',  ( -0.6146835312500006365, -14.06466310670085562, -2.385416667349463005 ) ) ;
#7148=CARTESIAN_POINT ( 'NONE',  ( 1.500000000000000222, -13.00000000000000533, -0.5625000013655934161 ) ) ;
#7156=CARTESIAN_POINT ( 'NONE',  ( -1.229367062500000163, -13.00000000000000533, -0.5937500006827968191 ) ) ;
#7167=DIRECTION ( 'NONE',  ( 0.000000000000000000, 0.000000000000000000, 1.000000000000000000 ) ) ;
#7173=PRODUCT_DEFINITION_CONTEXT ( 'detailed design', #10015, 'design' ) ;
#7174=CARTESIAN_POINT ( 'NONE',  ( -3.181725716174720498E-16, -14.73205080756888385, -1.625000000000000222 ) ) ;
#7182=DIRECTION ( 'NONE',  ( 0.8660254037844402619, -0.000000000000000000, 0.4999999999999972244 ) ) ;
#7185=( BOUNDED_CURVE ( )  B_SPLINE_CURVE ( 2, ( #2179, #6197, #5457, #5402, #8804, #7097, #8646 ),
 .UNSPECIFIED., .F., .T. ) 
 B_SPLINE_CURVE_WITH_KNOTS ( ( 3, 2, 2, 3 ),
 ( 0.5833333333333332593, 0.6111111111111110494, 0.6388888888888888395, 0.6666666666666666297 ),
 .UNSPECIFIED. ) 
 CURVE ( )  GEOMETRIC_REPRESENTATION_ITEM ( )  RATIONAL_B_SPLINE_CURVE ( ( 1.000000000000000444, 0.8660254037844381525, 1.000000000000000000, 0.8660254037844387076, 1.000000000000000000, 0.8660254037844387076, 1.000000000000000000 ) ) 
 REPRESENTATION_ITEM ( '' )  );
#7201=CARTESIAN_POINT ( 'NONE',  ( -1.500000000000000222, -13.00000000000000533, -0.3125000013655936937 ) ) ;
#7204=CARTESIAN_POINT ( 'NONE',  ( 1.229367062500000163, -13.00000000000000533, -2.781250000682796486 ) ) ;
#7210=LINE ( 'NONE', #4128, #3732 ) ;
#7225=ORIENTED_EDGE ( 'NONE', *, *, #9880, .T. ) ;
#7226=DIRECTION ( 'NONE',  ( 1.000000000000000000, 0.000000000000000000, 0.000000000000000000 ) ) ;
#7228=DIRECTION ( 'NONE',  ( 1.000000000000000000, 0.000000000000000000, 0.000000000000000000 ) ) ;
#7232=CARTESIAN_POINT ( 'NONE',  ( 1.500000000000000000, -13.86602540378444459, -0.5416666666666668517 ) ) ;
#7244=FILL_AREA_STYLE ('',( #7300 ) ) ;
#7248=( BOUNDED_CURVE ( )  B_SPLINE_CURVE ( 2, ( #9341, #534, #6834, #4604, #2817, #7845, #1974 ),
 .UNSPECIFIED., .F., .F. ) 
 B_SPLINE_CURVE_WITH_KNOTS ( ( 3, 2, 2, 3 ),
 ( 0.9166666666666666297, 0.9444444444444444198, 0.9722222222222222099, 1.000000000000000000 ),
 .UNSPECIFIED. ) 
 CURVE ( )  GEOMETRIC_REPRESENTATION_ITEM ( )  RATIONAL_B_SPLINE_CURVE ( ( 1.000000000000000000, 0.8660254037844387076, 1.000000000000000000, 0.8660254037844387076, 1.000000000000000000, 0.8660254037844387076, 1.000000000000000000 ) ) 
 REPRESENTATION_ITEM ( '' )  );
#7253=CARTESIAN_POINT ( 'NONE',  ( 1.500000000000000000, -13.86602540378444459, -1.604166668032260379 ) ) ;
#7284=CARTESIAN_POINT ( 'NONE',  ( -0.7500000000000007772, -14.29903810567666156, -0.6666666666666669627 ) ) ;
#7292=AXIS2_PLACEMENT_3D ( 'NONE', #8971, #758, #10477 ) ;
#7297=VECTOR ( 'NONE', #7368, 1000.000000000000000 ) ;
#7300=FILL_AREA_STYLE_COLOUR ( '', #10076 ) ;
#7311=CARTESIAN_POINT ( 'NONE',  ( 1.229367062500000385, -12.29022459553277002, -2.677083334016129967 ) ) ;
#7323=CARTESIAN_POINT ( 'NONE',  ( 1.229367062500000163, -13.00000000000000533, -0.3437500006827965970 ) ) ;
#7338=CARTESIAN_POINT ( 'NONE',  ( 8.692241771943170539E-17, -11.58044919106553650, -2.093750000682796486 ) ) ;
#7340=ADVANCED_FACE ( 'NONE', ( #10465 ), #4707, .T. ) ;
#7346=ORIENTED_EDGE ( 'NONE', *, *, #1899, .F. ) ;
#7353=EDGE_CURVE ( 'NONE', #6335, #8200, #8284, .T. ) ;
#7364=CARTESIAN_POINT ( 'NONE',  ( -0.7500000000000007772, -14.29903810567666156, -0.7291666680322601568 ) ) ;
#7368=DIRECTION ( 'NONE',  ( -0.000000000000000000, -0.000000000000000000, -1.000000000000000000 ) ) ;
#7381=DIRECTION ( 'NONE',  ( -1.000000000000000000, 0.000000000000000000, 0.000000000000000000 ) ) ;
#7392=ORIENTED_EDGE ( 'NONE', *, *, #8678, .T. ) ;
#7405=LINE ( 'NONE', #8315, #2294 ) ;
#7416=DIRECTION ( 'NONE',  ( 1.000000000000000000, 0.000000000000000000, 0.000000000000000000 ) ) ;
#7420=CARTESIAN_POINT ( 'NONE',  ( 0.6146835312499993043, -14.06466310670085562, -0.4270833340161298564 ) ) ;
#7423=DIRECTION ( 'NONE',  ( 0.000000000000000000, 0.000000000000000000, 1.000000000000000000 ) ) ;
#7431=VECTOR ( 'NONE', #4801, 1000.000000000000000 ) ;
#7437=ADVANCED_FACE ( 'NONE', ( #904 ), #8332, .T. ) ;
#7441=EDGE_LOOP ( 'NONE', ( #6701, #10071, #2723, #1202 ) ) ;
#7460=DIRECTION ( 'NONE',  ( 0.000000000000000000, 0.000000000000000000, 1.000000000000000000 ) ) ;
#7463=CARTESIAN_POINT ( 'NONE',  ( 1.060575238724907038E-16, -11.26794919243112680, -0.3750000000000002776 ) ) ;
#7471=CARTESIAN_POINT ( 'NONE',  ( 1.229367062500000163, -13.00000000000000533, -1.218750000682796486 ) ) ;
#7482=CARTESIAN_POINT ( 'NONE',  ( -0.6146835312500006365, -14.06466310670085562, -2.010416667349463005 ) ) ;
#7487=DIRECTION ( 'NONE',  ( 0.000000000000000000, 0.000000000000000000, 1.000000000000000000 ) ) ;
#7492=PLANE ( 'NONE',  #3544 ) ;
#7494=CARTESIAN_POINT ( 'NONE',  ( -0.6146835312500006365, -14.06466310670085562, -1.385416667349463227 ) ) ;
#7501=EDGE_CURVE ( 'NONE', #10421, #4827, #6839, .T. ) ;
#7506=ORIENTED_EDGE ( 'NONE', *, *, #2607, .T. ) ;
#7508=CARTESIAN_POINT ( 'NONE',  ( 0.6146835312500001924, -11.93533689329915326, -2.260416667349463449 ) ) ;
#7515=ORIENTED_EDGE ( 'NONE', *, *, #7866, .T. ) ;
#7520=CARTESIAN_POINT ( 'NONE',  ( -1.229367062500000163, -13.00000000000000533, 0.03124999931720332663 ) ) ;
#7527=CARTESIAN_POINT ( 'NONE',  ( 0.6146835312500001924, -11.93533689329915326, -1.760416667349463449 ) ) ;
#7531=EDGE_CURVE ( 'NONE', #1639, #7636, #268, .T. ) ;
#7539=CARTESIAN_POINT ( 'NONE',  ( 0.7500000000000003331, -11.70096189432334732, -1.979166668032260157 ) ) ;
#7543=CARTESIAN_POINT ( 'NONE',  ( 8.692241771943169307E-17, -11.58044919106553294, -1.593750000682796486 ) ) ;
#7547=CARTESIAN_POINT ( 'NONE',  ( 1.229367062500000163, -12.29022459553277002, -2.177083334016129523 ) ) ;
#7549=EDGE_LOOP ( 'NONE', ( #3530, #6380, #5504, #6204 ) ) ;
#7554=ORIENTED_EDGE ( 'NONE', *, *, #1450, .F. ) ;
#7569=CARTESIAN_POINT ( 'NONE',  ( -1.229367062500000163, -12.29022459553277002, -1.510416667349463227 ) ) ;
#7571=CARTESIAN_POINT ( 'NONE',  ( 1.500000000000000222, -13.00000000000000533, -3.000000000000000000 ) ) ;
#7572=CARTESIAN_POINT ( 'NONE',  ( -0.7499999999999997780, -11.70096189432334555, -0.8958333346989268975 ) ) ;
#7577=CARTESIAN_POINT ( 'NONE',  ( 0.6146835312500001924, -11.93533689329915326, -0.2604166673494633377 ) ) ;
#7585=ADVANCED_FACE ( 'NONE', ( #4538 ), #2065, .T. ) ;
#7590=( BOUNDED_SURFACE ( )  B_SPLINE_SURFACE ( 1, 2, ( 
 ( #8538, #10137, #10238, #2172, #9496, #3701, #3073, #2858, #9336, #10289, #2072, #8636, #2917, #2228, #8688, #1424, #3860, #7088, #10345, #6292, #9548, #3174, #4701, #7253, #9602, #4921, #8950, #3972, #1644, #8168, #898, #6399, #3122, #9655, #6455, #4124, #8904, #2492, #7947, #10402, #4866, #9712, #8852, #10498, #7364, #4024, #8111, #3282, #106, #794, #2383, #3226, #740, #5704, #7201, #844, #5609, #3334, #1594, #9763, #2439, #8008, #685, #53, #4817, #5659, #4075, #3918, #1695, #6349, #5501, #1538, #8063 ),
 ( #10457, #7311, #6505, #2330, #6559, #9811, #8743, #1479, #7143, #5552, #8795, #4765, #366, #3385, #5124, #6613, #2692, #2749, #4227, #6816, #5911, #9168, #9867, #9214, #1800, #4177, #6711, #1101, #3536, #7569, #1054, #5073, #8372, #263, #6761, #8327, #7471, #5177, #5809, #2595, #9917, #9062, #1954, #9113, #9008, #6659, #5960, #2541, #1905, #5760, #5027, #8271, #997, #3590, #9969, #2646, #4972, #212, #4326, #10024, #3436, #1745, #4275, #312, #5861, #1849, #7520, #8425, #3490, #1151, #4375, #7621, #8218 ) ),
 .UNSPECIFIED., .F., .F., .F. ) 
 B_SPLINE_SURFACE_WITH_KNOTS ( ( 2, 2 ),
 ( 3, 2, 2, 2, 2, 2, 2, 2, 2, 2, 2, 2, 2, 2, 2, 2, 2, 2, 2, 2, 2, 2, 2, 2, 2, 2, 2, 2, 2, 2, 2, 2, 2, 2, 2, 2, 3 ),
 ( 0.000000000000000000, 1.000000000000000000 ),
 ( 0.000000000000000000, 0.02777777777777777624, 0.05555555555555555247, 0.08333333333333332871, 0.1111111111111111049, 0.1388888888888888951, 0.1666666666666666574, 0.1944444444444444475, 0.2222222222222222099, 0.2500000000000000000, 0.2777777777777777901, 0.3055555555555555802, 0.3333333333333333148, 0.3611111111111111049, 0.3888888888888888951, 0.4166666666666666852, 0.4444444444444444198, 0.4722222222222222099, 0.5000000000000000000, 0.5277777777777777901, 0.5555555555555555802, 0.5833333333333333703, 0.6111111111111111605, 0.6388888888888888395, 0.6666666666666666297, 0.6944444444444444198, 0.7222222222222222099, 0.7500000000000000000, 0.7777777777777777901, 0.8055555555555555802, 0.8333333333333333703, 0.8611111111111111605, 0.8888888888888888395, 0.9166666666666666297, 0.9444444444444444198, 0.9722222222222222099, 1.000000000000000000 ),
 .UNSPECIFIED. ) 
 GEOMETRIC_REPRESENTATION_ITEM ( )  RATIONAL_B_SPLINE_SURFACE ( (
 ( 1.000000000000000000, 0.8660254037844387076, 1.000000000000000000, 0.8660254037844387076, 1.000000000000000000, 0.8660254037844387076, 1.000000000000000000, 0.8660254037844387076, 1.000000000000000000, 0.8660254037844387076, 1.000000000000000000, 0.8660254037844387076, 1.000000000000000000, 0.8660254037844387076, 1.000000000000000000, 0.8660254037844387076, 1.000000000000000000, 0.8660254037844387076, 1.000000000000000000, 0.8660254037844387076, 1.000000000000000000, 0.8660254037844387076, 1.000000000000000000, 0.8660254037844387076, 1.000000000000000000, 0.8660254037844387076, 1.000000000000000000, 0.8660254037844387076, 1.000000000000000000, 0.8660254037844387076, 1.000000000000000000, 0.8660254037844387076, 1.000000000000000000, 0.8660254037844387076, 1.000000000000000000, 0.8660254037844387076, 1.000000000000000000, 0.8660254037844387076, 1.000000000000000000, 0.8660254037844387076, 1.000000000000000000, 0.8660254037844387076, 1.000000000000000000, 0.8660254037844387076, 1.000000000000000000, 0.8660254037844387076, 1.000000000000000000, 0.8660254037844387076, 1.000000000000000000, 0.8660254037844387076, 1.000000000000000000, 0.8660254037844387076, 1.000000000000000000, 0.8660254037844387076, 1.000000000000000000, 0.8660254037844387076, 1.000000000000000000, 0.8660254037844387076, 1.000000000000000000, 0.8660254037844387076, 1.000000000000000000, 0.8660254037844387076, 1.000000000000000000, 0.8660254037844387076, 1.000000000000000000, 0.8660254037844387076, 1.000000000000000000, 0.8660254037844387076, 1.000000000000000000, 0.8660254037844387076, 1.000000000000000000, 0.8660254037844387076, 1.000000000000000000),
 ( 1.000000000000000000, 0.8660254037844387076, 1.000000000000000000, 0.8660254037844387076, 1.000000000000000000, 0.8660254037844387076, 1.000000000000000000, 0.8660254037844387076, 1.000000000000000000, 0.8660254037844387076, 1.000000000000000000, 0.8660254037844387076, 1.000000000000000000, 0.8660254037844387076, 1.000000000000000000, 0.8660254037844387076, 1.000000000000000000, 0.8660254037844387076, 1.000000000000000000, 0.8660254037844387076, 1.000000000000000000, 0.8660254037844387076, 1.000000000000000000, 0.8660254037844387076, 1.000000000000000000, 0.8660254037844387076, 1.000000000000000000, 0.8660254037844387076, 1.000000000000000000, 0.8660254037844387076, 1.000000000000000000, 0.8660254037844387076, 1.000000000000000000, 0.8660254037844387076, 1.000000000000000000, 0.8660254037844387076, 1.000000000000000000, 0.8660254037844387076, 1.000000000000000000, 0.8660254037844387076, 1.000000000000000000, 0.8660254037844387076, 1.000000000000000000, 0.8660254037844387076, 1.000000000000000000, 0.8660254037844387076, 1.000000000000000000, 0.8660254037844387076, 1.000000000000000000, 0.8660254037844387076, 1.000000000000000000, 0.8660254037844387076, 1.000000000000000000, 0.8660254037844387076, 1.000000000000000000, 0.8660254037844387076, 1.000000000000000000, 0.8660254037844387076, 1.000000000000000000, 0.8660254037844387076, 1.000000000000000000, 0.8660254037844387076, 1.000000000000000000, 0.8660254037844387076, 1.000000000000000000, 0.8660254037844387076, 1.000000000000000000, 0.8660254037844387076, 1.000000000000000000, 0.8660254037844387076, 1.000000000000000000, 0.8660254037844387076, 1.000000000000000000) ) ) 
 REPRESENTATION_ITEM ( '' )  SURFACE ( )  );
#7591=CARTESIAN_POINT ( 'NONE',  ( -0.6146835312499998594, -11.93533689329915326, -1.052083334016129967 ) ) ;
#7593=CARTESIAN_POINT ( 'NONE',  ( 1.229367062500000163, -13.00000000000000533, -1.218750000682796486 ) ) ;
#7606=CARTESIAN_POINT ( 'NONE',  ( -1.229367062500000163, -13.00000000000000533, -0.09375000068279679133 ) ) ;
#7620=ORIENTED_EDGE ( 'NONE', *, *, #1835, .F. ) ;
#7621=CARTESIAN_POINT ( 'NONE',  ( 1.229367062499999719, -13.70977540446724063, 0.2395833326505366900 ) ) ;
#7622=VECTOR ( 'NONE', #4581, 999.9999999999998863 ) ;
#7633=CARTESIAN_POINT ( 'NONE',  ( 8.692241771943170539E-17, -11.58044919106553650, -1.218750000682796930 ) ) ;
#7636=VERTEX_POINT ( 'NONE', #6978 ) ;
#7638=AXIS2_PLACEMENT_3D ( 'NONE', #5924, #7423, #276 ) ;
#7646=CARTESIAN_POINT ( 'NONE',  ( 1.500000000000000222, -13.00000000000000533, -2.062500001365593416 ) ) ;
#7649=CARTESIAN_POINT ( 'NONE',  ( 1.229367062499999719, -13.70977540446724063, -1.760416667349463227 ) ) ;
#7651=CARTESIAN_POINT ( 'NONE',  ( -2.607672531582950546E-16, -14.41955080893447416, 0.1562499993172034307 ) ) ;
#7656=ORIENTED_EDGE ( 'NONE', *, *, #3375, .F. ) ;
#7661=CARTESIAN_POINT ( 'NONE',  ( -1.229367062500000385, -13.70977540446723886, -1.052083334016129967 ) ) ;
#7663=ORIENTED_EDGE ( 'NONE', *, *, #828, .T. ) ;
#7677=UNCERTAINTY_MEASURE_WITH_UNIT (LENGTH_MEASURE( 1.000000000000000082E-05 ), #8562, 'distance_accuracy_value', 'NONE');
#7711=DIRECTION ( 'NONE',  ( 0.000000000000000000, 0.000000000000000000, 1.000000000000000000 ) ) ;
#7714=ADVANCED_FACE ( 'NONE', ( #5339 ), #8582, .T. ) ;
#7717=CARTESIAN_POINT ( 'NONE',  ( -1.229367062500000163, -12.29022459553277002, -1.135416667349463227 ) ) ;
#7718=ORIENTED_EDGE ( 'NONE', *, *, #5222, .F. ) ;
#7721=CARTESIAN_POINT ( 'NONE',  ( 1.500000000000000222, -13.00000000000000533, -2.500000000000000000 ) ) ;
#7725=EDGE_LOOP ( 'NONE', ( #2309, #8487, #45 ) ) ;
#7732=CARTESIAN_POINT ( 'NONE',  ( 0.7500000000000003331, -11.70096189432334732, -1.479166668032260157 ) ) ;
#7746=PRODUCT ( 'position sensor magnet', 'position sensor magnet', '', ( #8704 ) ) ;
#7753=CARTESIAN_POINT ( 'NONE',  ( 1.229367062500000385, -12.29022459553277002, -2.302083334016129967 ) ) ;
#7755=CARTESIAN_POINT ( 'NONE',  ( 0.6146835312499993043, -14.06466310670085562, -0.8020833340161299674 ) ) ;
#7762=CARTESIAN_POINT ( 'NONE',  ( -1.500000000000000222, -13.00000000000000533, -0.3125000013655936937 ) ) ;
#7766=CARTESIAN_POINT ( 'NONE',  ( 1.229367062500000385, -12.29022459553277002, -1.802083334016129967 ) ) ;
#7776=ORIENTED_EDGE ( 'NONE', *, *, #5222, .T. ) ;
#7780=ORIENTED_EDGE ( 'NONE', *, *, #3812, .T. ) ;
#7781=EDGE_CURVE ( 'NONE', #6751, #5863, #4808, .T. ) ;
#7796=EDGE_CURVE ( 'NONE', #2259, #6255, #4695, .T. ) ;
#7806=CARTESIAN_POINT ( 'NONE',  ( 0.6146835312500001924, -11.93533689329915326, -2.760416667349463449 ) ) ;
#7811=CARTESIAN_POINT ( 'NONE',  ( 0.6146835312500001924, -11.93533689329915326, -0.1354166673494631989 ) ) ;
#7818=CARTESIAN_POINT ( 'NONE',  ( -0.7500000000000007772, -14.29903810567666156, -1.666666666666666741 ) ) ;
#7823=CARTESIAN_POINT ( 'NONE',  ( 1.229367062499999719, -13.70977540446724063, -1.385416667349463671 ) ) ;
#7835=DIRECTION ( 'NONE',  ( 1.000000000000000000, 0.000000000000000000, -0.000000000000000000 ) ) ;
#7836=ORIENTED_EDGE ( 'NONE', *, *, #9693, .F. ) ;
#7845=CARTESIAN_POINT ( 'NONE',  ( 1.499999999999999778, -13.86602540378444637, -0.04166666666666685170 ) ) ;
#7854=CARTESIAN_POINT ( 'NONE',  ( -1.229367062500000163, -12.29022459553277002, -2.635416667349463449 ) ) ;
#7860=CARTESIAN_POINT ( 'NONE',  ( -1.500000000000000222, -13.00000000000000533, -2.312500001365593860 ) ) ;
#7864=DIRECTION ( 'NONE',  ( 0.000000000000000000, 0.000000000000000000, 1.000000000000000000 ) ) ;
#7866=EDGE_CURVE ( 'NONE', #8200, #6255, #1836, .T. ) ;
#7867=CARTESIAN_POINT ( 'NONE',  ( -3.181725716174720991E-16, -14.73205080756888563, -0.1875000013655935827 ) ) ;
#7875=CARTESIAN_POINT ( 'NONE',  ( 0.7500000000000003331, -11.70096189432334732, -0.9166666666666667407 ) ) ;
#7883=CARTESIAN_POINT ( 'NONE',  ( -1.499999999999998224, -12.13397459621556607, -1.354166668032260379 ) ) ;
#7904=CARTESIAN_POINT ( 'NONE',  ( -1.499999999999996891, -12.13397459621556429, -2.291666666666666519 ) ) ;
#7908=CARTESIAN_POINT ( 'NONE',  ( -1.229367062500000163, -12.29022459553277002, -2.135416667349463449 ) ) ;
#7910=FACE_OUTER_BOUND ( 'NONE', #4160, .T. ) ;
#7924=CARTESIAN_POINT ( 'NONE',  ( 1.500000000000000444, -12.13397459621556607, -0.4583333333333336479 ) ) ;
#7928=DIRECTION ( 'NONE',  ( 1.000000000000000000, 0.000000000000000000, 0.000000000000000000 ) ) ;
#7947=CARTESIAN_POINT ( 'NONE',  ( 0.7500000000000003331, -11.70096189432334732, -0.9791666680322602678 ) ) ;
#7949=CARTESIAN_POINT ( 'NONE',  ( 1.060575238724907038E-16, -11.26794919243112680, -0.4375000013655938602 ) ) ;
#7956=CLOSED_SHELL ( 'NONE', ( #5732, #9997, #107, #7437, #5046, #797, #7994, #5553, #2641, #148, #7585, #3405, #7340, #3188, #3964, #6872, #7714, #10039, #2351, #161, #9083, #9749, #1341, #1765 ) ) ;
#7957=DIRECTION ( 'NONE',  ( 0.000000000000000000, 0.000000000000000000, 1.000000000000000000 ) ) ;
#7960=VECTOR ( 'NONE', #3168, 1000.000000000000000 ) ;
#7963=CARTESIAN_POINT ( 'NONE',  ( 0.6146835312500001924, -11.93533689329915326, -1.260416667349463227 ) ) ;
#7968=ORIENTED_EDGE ( 'NONE', *, *, #10325, .F. ) ;
#7972=CARTESIAN_POINT ( 'NONE',  ( -3.181725716174720991E-16, -14.73205080756888563, -1.687500001365593638 ) ) ;
#7981=EDGE_CURVE ( 'NONE', #2223, #7636, #2919, .T. ) ;
#7984=CARTESIAN_POINT ( 'NONE',  ( 0.7500000000000003331, -11.70096189432334732, -0.4166666666666667407 ) ) ;
#7987=ORIENTED_EDGE ( 'NONE', *, *, #8671, .T. ) ;
#7988=CARTESIAN_POINT ( 'NONE',  ( -1.499999999999999778, -12.13397459621556784, -0.7916666666666666297 ) ) ;
#7991=CARTESIAN_POINT ( 'NONE',  ( 0.6146835312499993043, -14.06466310670085562, 0.07291666598386974119 ) ) ;
#7993=EDGE_LOOP ( 'NONE', ( #884, #8307 ) ) ;
#7994=ADVANCED_FACE ( 'NONE', ( #3482 ), #206, .T. ) ;
#8008=CARTESIAN_POINT ( 'NONE',  ( 1.500000000000000444, -12.13397459621556607, -0.02083333469892703974 ) ) ;
#8014=DIRECTION ( 'NONE',  ( 0.000000000000000000, 0.000000000000000000, 1.000000000000000000 ) ) ;
#8020=CARTESIAN_POINT ( 'NONE',  ( -2.607672531582950546E-16, -14.41955080893447416, -0.4687500006827967081 ) ) ;
#8031=EDGE_CURVE ( 'NONE', #10270, #8600, #4425, .T. ) ;
#8038=CARTESIAN_POINT ( 'NONE',  ( 0.7500000000000003331, -11.70096189432334732, -1.416666666666666741 ) ) ;
#8041=ORIENTED_EDGE ( 'NONE', *, *, #8700, .T. ) ;
#8058=ORIENTED_EDGE ( 'NONE', *, *, #6377, .T. ) ;
#8063=CARTESIAN_POINT ( 'NONE',  ( 1.500000000000000222, -13.00000000000000533, 0.4374999986344065284 ) ) ;
#8070=CARTESIAN_POINT ( 'NONE',  ( -3.181725716174720991E-16, -14.73205080756888563, -2.125000000000000000 ) ) ;
#8087=CARTESIAN_POINT ( 'NONE',  ( 1.500000000000000444, -12.13397459621556607, -2.458333333333333037 ) ) ;
#8105=CARTESIAN_POINT ( 'NONE',  ( -0.7499999999999997780, -11.70096189432334555, -1.833333333333333481 ) ) ;
#8111=CARTESIAN_POINT ( 'NONE',  ( 0.7499999999999991118, -14.29903810567666333, -0.6458333346989268975 ) ) ;
#8116=DIRECTION ( 'NONE',  ( -0.000000000000000000, -0.000000000000000000, -1.000000000000000000 ) ) ;
#8124=CARTESIAN_POINT ( 'NONE',  ( -0.6146835312499998594, -11.93533689329915326, -1.177083334016129967 ) ) ;
#8168=CARTESIAN_POINT ( 'NONE',  ( -1.500000000000000000, -12.13397459621556607, -1.354166668032260157 ) ) ;
#8173=CARTESIAN_POINT ( 'NONE',  ( 0.000000000000000000, -13.00000000000000533, -3.000000000000000000 ) ) ;
#8175=CARTESIAN_POINT ( 'NONE',  ( 1.229367062500000163, -13.00000000000000533, -2.843750000682796486 ) ) ;
#8180=PLANE ( 'NONE',  #6307 ) ;
#8200=VERTEX_POINT ( 'NONE', #8834 ) ;
#8218=CARTESIAN_POINT ( 'NONE',  ( 1.229367062500000163, -13.00000000000000533, 0.2812499993172035695 ) ) ;
#8223=CARTESIAN_POINT ( 'NONE',  ( 0.000000000000000000, -13.00000000000000533, -3.000000000000000000 ) ) ;
#8227=AXIS2_PLACEMENT_3D ( 'NONE', #6652, #7460, #5903 ) ;
#8228=CARTESIAN_POINT ( 'NONE',  ( -0.6146835312499998594, -11.93533689329915326, -2.177083334016129967 ) ) ;
#8232=CARTESIAN_POINT ( 'NONE',  ( -0.6146835312500006365, -14.06466310670085562, -0.01041666734946352160 ) ) ;
#8243=DIRECTION ( 'NONE',  ( 0.000000000000000000, 0.000000000000000000, 1.000000000000000000 ) ) ;
#8249=EDGE_CURVE ( 'NONE', #8955, #5062, #4331, .T. ) ;
#8271=CARTESIAN_POINT ( 'NONE',  ( 8.692241771943169307E-17, -11.58044919106553294, -0.5937500006827968191 ) ) ;
#8280=CARTESIAN_POINT ( 'NONE',  ( -1.229367062500000163, -13.00000000000000533, -1.093750000682796486 ) ) ;
#8284=( BOUNDED_CURVE ( )  B_SPLINE_CURVE ( 2, ( #3865, #10353, #8749, #8070, #4029, #1600, #9557 ),
 .UNSPECIFIED., .F., .T. ) 
 B_SPLINE_CURVE_WITH_KNOTS ( ( 3, 2, 2, 3 ),
 ( 0.2499999999999999167, 0.2777777777777777346, 0.3055555555555555802, 0.3333333333333333148 ),
 .UNSPECIFIED. ) 
 CURVE ( )  GEOMETRIC_REPRESENTATION_ITEM ( )  RATIONAL_B_SPLINE_CURVE ( ( 1.000000000000000222, 0.8660254037844382635, 1.000000000000000000, 0.8660254037844387076, 1.000000000000000000, 0.8660254037844387076, 1.000000000000000000 ) ) 
 REPRESENTATION_ITEM ( '' )  );
#8294=CARTESIAN_POINT ( 'NONE',  ( -0.6146835312499998594, -11.93533689329915326, -1.552083334016129967 ) ) ;
#8307=ORIENTED_EDGE ( 'NONE', *, *, #5401, .T. ) ;
#8310=CARTESIAN_POINT ( 'NONE',  ( 1.229367062499999719, -13.70977540446724063, -2.385416667349463005 ) ) ;
#8315=CARTESIAN_POINT ( 'NONE',  ( 1.500000000000000222, -13.00000000000000533, -3.000000000000000000 ) ) ;
#8327=CARTESIAN_POINT ( 'NONE',  ( 1.229367062499999719, -13.70977540446724063, -1.260416667349463449 ) ) ;
#8332=CYLINDRICAL_SURFACE ( 'NONE', #6929, 1.500000000000000222 ) ;
#8336=CARTESIAN_POINT ( 'NONE',  ( 0.6146835312500001924, -11.93533689329915326, -0.7604166673494633377 ) ) ;
#8345=DIRECTION ( 'NONE',  ( 0.000000000000000000, -0.000000000000000000, -1.000000000000000000 ) ) ;
#8350=CARTESIAN_POINT ( 'NONE',  ( -2.607672531582950546E-16, -14.41955080893447416, -2.343750000682796042 ) ) ;
#8355=VERTEX_POINT ( 'NONE', #9897 ) ;
#8372=CARTESIAN_POINT ( 'NONE',  ( -0.6146835312500006365, -14.06466310670085562, -1.385416667349463227 ) ) ;
#8378=CARTESIAN_POINT ( 'NONE',  ( 0.000000000000000000, -13.00000000000000533, -3.000000000000000000 ) ) ;
#8382=CARTESIAN_POINT ( 'NONE',  ( 1.229367062500000163, -12.29022459553277002, -0.3020833340161301339 ) ) ;
#8394=CARTESIAN_POINT ( 'NONE',  ( -1.500000000000000222, -13.00000000000000533, -1.812500001365593416 ) ) ;
#8397=CARTESIAN_POINT ( 'NONE',  ( 0.6146835312500001924, -11.93533689329915326, -2.635416667349463449 ) ) ;
#8401=CARTESIAN_POINT ( 'NONE',  ( -1.229367062500000163, -12.29022459553277002, -1.510416667349463227 ) ) ;
#8407=CARTESIAN_POINT ( 'NONE',  ( -1.500000000000000222, -13.00000000000000533, -3.000000000000000000 ) ) ;
#8419=CARTESIAN_POINT ( 'NONE',  ( 1.364683531250000303, -13.00000000000000533, -2.921875000341398465 ) ) ;
#8425=CARTESIAN_POINT ( 'NONE',  ( -1.229367062500000385, -13.70977540446723886, 0.07291666598387017140 ) ) ;
#8428=EDGE_LOOP ( 'NONE', ( #2349, #7225, #7663, #7968, #7656, #3800, #2630, #10221, #2831, #7836, #7620, #3859, #6322, #7718, #2967 ) ) ;
#8434=CARTESIAN_POINT ( 'NONE',  ( -0.6146835312500006365, -14.06466310670085562, -0.01041666734946352160 ) ) ;
#8440=DIRECTION ( 'NONE',  ( 1.000000000000000000, 0.000000000000000000, 0.000000000000000000 ) ) ;
#8449=CARTESIAN_POINT ( 'NONE',  ( 0.6146835312500001924, -11.93533689329915326, -0.6354166673494632267 ) ) ;
#8460=CARTESIAN_POINT ( 'NONE',  ( 1.229367062500000163, -13.00000000000000533, -0.3437500006827965970 ) ) ;
#8467=AXIS2_PLACEMENT_3D ( 'NONE', #9663, #8014, #9769 ) ;
#8469=ORIENTED_EDGE ( 'NONE', *, *, #5557, .T. ) ;
#8470=STYLED_ITEM ( 'NONE', ( #1294 ), #4775 ) ;
#8480=CARTESIAN_POINT ( 'NONE',  ( 0.000000000000000000, -13.00000000000000533, -3.000000000000000000 ) ) ;
#8487=ORIENTED_EDGE ( 'NONE', *, *, #940, .T. ) ;
#8492=CARTESIAN_POINT ( 'NONE',  ( -1.500000000000000222, -13.00000000000000533, -2.750000000000000000 ) ) ;
#8498=CARTESIAN_POINT ( 'NONE',  ( 0.6146835312499993043, -14.06466310670085562, -0.8020833340161299674 ) ) ;
#8500=CARTESIAN_POINT ( 'NONE',  ( -0.6146835312500006365, -14.06466310670085562, -0.3854166673494634487 ) ) ;
#8502=EDGE_CURVE ( 'NONE', #9020, #9003, #6044, .T. ) ;
#8512=CARTESIAN_POINT ( 'NONE',  ( 0.6146835312500001924, -11.93533689329915326, -0.2604166673494633377 ) ) ;
#8526=CARTESIAN_POINT ( 'NONE',  ( 0.7500000000000003331, -11.70096189432334732, -1.416666666666666741 ) ) ;
#8538=CARTESIAN_POINT ( 'NONE',  ( 1.500000000000000222, -13.00000000000000533, -2.562500001365593416 ) ) ;
#8545=CARTESIAN_POINT ( 'NONE',  ( 1.060575238724907038E-16, -11.26794919243112680, -1.937500001365593416 ) ) ;
#8548=CARTESIAN_POINT ( 'NONE',  ( -0.6146835312500006365, -14.06466310670085562, -2.510416667349463005 ) ) ;
#8562=( LENGTH_UNIT ( ) NAMED_UNIT ( * ) SI_UNIT ( .MILLI., .METRE. ) );
#8565=CARTESIAN_POINT ( 'NONE',  ( -1.229367062500000163, -13.00000000000000533, -1.093750000682796486 ) ) ;
#8582=PLANE ( 'NONE',  #4729 ) ;
#8592=CYLINDRICAL_SURFACE ( 'NONE', #8983, 1.500000000000000222 ) ;
#8597=CARTESIAN_POINT ( 'NONE',  ( 0.6146835312500001924, -11.93533689329915326, -0.1354166673494631989 ) ) ;
#8599=CARTESIAN_POINT ( 'NONE',  ( 0.6146835312499993043, -14.06466310670085562, 0.1979166659838698661 ) ) ;
#8600=VERTEX_POINT ( 'NONE', #2091 ) ;
#8606=SURFACE_STYLE_USAGE ( .BOTH. , #4571 ) ;
#8608=( BOUNDED_CURVE ( )  B_SPLINE_CURVE ( 2, ( #20, #2347, #8973, #7972, #3249, #3349, #1716 ),
 .UNSPECIFIED., .F., .T. ) 
 B_SPLINE_CURVE_WITH_KNOTS ( ( 3, 2, 2, 3 ),
 ( 0.2500000000000000000, 0.2777777777777777901, 0.3055555555555555802, 0.3333333333333333148 ),
 .UNSPECIFIED. ) 
 CURVE ( )  GEOMETRIC_REPRESENTATION_ITEM ( )  RATIONAL_B_SPLINE_CURVE ( ( 1.000000000000000000, 0.8660254037844387076, 1.000000000000000000, 0.8660254037844387076, 1.000000000000000000, 0.8660254037844387076, 1.000000000000000000 ) ) 
 REPRESENTATION_ITEM ( '' )  );
#8609=CARTESIAN_POINT ( 'NONE',  ( 1.229367062500000163, -13.00000000000000533, -1.843750000682796708 ) ) ;
#8629=CARTESIAN_POINT ( 'NONE',  ( 0.000000000000000000, -13.00000000000000533, 2.000000000000000000 ) ) ;
#8636=CARTESIAN_POINT ( 'NONE',  ( 1.500000000000000000, -13.86602540378444459, -2.104166668032260379 ) ) ;
#8641=FACE_OUTER_BOUND ( 'NONE', #5270, .T. ) ;
#8646=CARTESIAN_POINT ( 'NONE',  ( 1.500000000000000222, -13.00000000000000533, -1.000000000000000000 ) ) ;
#8650=CARTESIAN_POINT ( 'NONE',  ( 1.229367062500000163, -13.00000000000000533, -2.343750000682796486 ) ) ;
#8656=ORIENTED_EDGE ( 'NONE', *, *, #1835, .T. ) ;
#8666=CARTESIAN_POINT ( 'NONE',  ( 1.229367062499999719, -13.70977540446724063, -0.8854166673494634487 ) ) ;
#8669=DIRECTION ( 'NONE',  ( 0.000000000000000000, 0.000000000000000000, 1.000000000000000000 ) ) ;
#8671=EDGE_CURVE ( 'NONE', #1061, #2223, #2991, .T. ) ;
#8675=CARTESIAN_POINT ( 'NONE',  ( -1.499999999999996669, -12.13397459621556607, -1.291666666666667185 ) ) ;
#8678=EDGE_CURVE ( 'NONE', #6255, #8785, #1514, .T. ) ;
#8688=CARTESIAN_POINT ( 'NONE',  ( 0.7500000000000003331, -11.70096189432334732, -1.979166668032260157 ) ) ;
#8693=CARTESIAN_POINT ( 'NONE',  ( 0.7499999999999991118, -14.29903810567666333, -0.6458333346989268975 ) ) ;
#8699=CARTESIAN_POINT ( 'NONE',  ( -0.6146835312499998594, -11.93533689329915326, -0.05208333401612993963 ) ) ;
#8700=EDGE_CURVE ( 'NONE', #4078, #8200, #3881, .T. ) ;
#8702=CYLINDRICAL_SURFACE ( 'NONE', #10057, 1.500000000000000222 ) ;
#8704=PRODUCT_CONTEXT ( 'NONE', #4923, 'mechanical' ) ;
#8715=CARTESIAN_POINT ( 'NONE',  ( -1.500000000000000666, -13.86602540378444459, -1.208333333333333703 ) ) ;
#8720=CARTESIAN_POINT ( 'NONE',  ( 1.500000000000000222, -13.00000000000000533, -2.562500001365593416 ) ) ;
#8723=CARTESIAN_POINT ( 'NONE',  ( 1.364683531250000303, -13.00000000000000533, 0.3593749989758050489 ) ) ;
#8743=CARTESIAN_POINT ( 'NONE',  ( -1.229367062500000163, -13.00000000000000533, -2.468750000682796486 ) ) ;
#8748=CARTESIAN_POINT ( 'NONE',  ( -1.500000000000000222, -13.00000000000000533, -2.312500001365593860 ) ) ;
#8749=CARTESIAN_POINT ( 'NONE',  ( -0.7500000000000007772, -14.29903810567666156, -2.166666666666666519 ) ) ;
#8753=CARTESIAN_POINT ( 'NONE',  ( 1.229367062500000163, -13.00000000000000533, -1.343750000682796486 ) ) ;
#8759=FACE_OUTER_BOUND ( 'NONE', #7441, .T. ) ;
#8762=FACE_OUTER_BOUND ( 'NONE', #9873, .T. ) ;
#8767=CARTESIAN_POINT ( 'NONE',  ( -1.500000000000000666, -13.86602540378444637, -0.2708333346989268420 ) ) ;
#8770=CARTESIAN_POINT ( 'NONE',  ( -1.500000000000000222, -13.00000000000000533, -0.7500000000000002220 ) ) ;
#8784=( NAMED_UNIT ( * ) PLANE_ANGLE_UNIT ( ) SI_UNIT ( $, .RADIAN. ) );
#8785=VERTEX_POINT ( 'NONE', #6421 ) ;
#8795=CARTESIAN_POINT ( 'NONE',  ( 0.6146835312499993043, -14.06466310670085562, -2.302083334016129967 ) ) ;
#8804=CARTESIAN_POINT ( 'NONE',  ( 0.7499999999999991118, -14.29903810567666333, -1.083333333333333481 ) ) ;
#8809=CARTESIAN_POINT ( 'NONE',  ( 1.229367062500000163, -13.00000000000000533, 0.1562499993172034307 ) ) ;
#8828=CARTESIAN_POINT ( 'NONE',  ( 1.500000000000000444, -12.13397459621556607, -1.958333333333333481 ) ) ;
#8834=CARTESIAN_POINT ( 'NONE',  ( 1.500000000000000222, -13.00000000000000533, -2.000000000000000000 ) ) ;
#8836=CARTESIAN_POINT ( 'NONE',  ( 1.500000000000000222, -13.00000000000000533, -3.000000000000000000 ) ) ;
#8852=CARTESIAN_POINT ( 'NONE',  ( -1.500000000000000222, -13.00000000000000533, -0.8125000013655935271 ) ) ;
#8864=CARTESIAN_POINT ( 'NONE',  ( -1.229367062500000163, -13.00000000000000533, -1.093750000682796486 ) ) ;
#8879=CARTESIAN_POINT ( 'NONE',  ( -0.7499999999999997780, -11.70096189432334555, -1.333333333333333481 ) ) ;
#8892=VERTEX_POINT ( 'NONE', #3598 ) ;
#8893=AXIS2_PLACEMENT_3D ( 'NONE', #10407, #8116, #2390 ) ;
#8904=CARTESIAN_POINT ( 'NONE',  ( 1.500000000000000222, -13.00000000000000533, -1.062500001365593416 ) ) ;
#8916=CARTESIAN_POINT ( 'NONE',  ( 1.500000000000000222, -13.00000000000000533, -1.000000000000000000 ) ) ;
#8917=ADVANCED_BREP_SHAPE_REPRESENTATION ( '', ( #4775, #2101 ), #581 ) ;
#8928=DIRECTION ( 'NONE',  ( 1.000000000000000000, 0.000000000000000000, 0.000000000000000000 ) ) ;
#8940=PRESENTATION_STYLE_ASSIGNMENT (( #3215 ) ) ;
#8950=CARTESIAN_POINT ( 'NONE',  ( 0.7500000000000003331, -11.70096189432334732, -1.479166668032260157 ) ) ;
#8955=VERTEX_POINT ( 'NONE', #3545 ) ;
#8962=ORIENTED_EDGE ( 'NONE', *, *, #6432, .F. ) ;
#8964=CARTESIAN_POINT ( 'NONE',  ( 1.229367062499999719, -13.70977540446724063, 0.1145833326505365929 ) ) ;
#8968=FACE_OUTER_BOUND ( 'NONE', #1511, .T. ) ;
#8971=CARTESIAN_POINT ( 'NONE',  ( 0.000000000000000000, -13.00000000000000533, 0.000000000000000000 ) ) ;
#8973=CARTESIAN_POINT ( 'NONE',  ( -0.7500000000000007772, -14.29903810567666156, -1.729166668032260157 ) ) ;
#8983=AXIS2_PLACEMENT_3D ( 'NONE', #4657, #7957, #6194 ) ;
#8997=CARTESIAN_POINT ( 'NONE',  ( 1.229367062500000163, -13.00000000000000533, -2.843750000682796486 ) ) ;
#9003=VERTEX_POINT ( 'NONE', #2168 ) ;
#9007=EDGE_LOOP ( 'NONE', ( #2155, #1931, #4593, #2954 ) ) ;
#9008=CARTESIAN_POINT ( 'NONE',  ( -0.6146835312500006365, -14.06466310670085562, -0.8854166673494632267 ) ) ;
#9013=CARTESIAN_POINT ( 'NONE',  ( -1.500000000000000222, -13.00000000000000533, -1.812500001365593416 ) ) ;
#9017=CARTESIAN_POINT ( 'NONE',  ( 1.229367062500000163, -13.70977540446723886, -2.385416667349463005 ) ) ;
#9020=VERTEX_POINT ( 'NONE', #3802 ) ;
#9023=( BOUNDED_CURVE ( )  B_SPLINE_CURVE ( 2, ( #10090, #10241, #5349, #5195, #6031, #9283, #8492 ),
 .UNSPECIFIED., .F., .T. ) 
 B_SPLINE_CURVE_WITH_KNOTS ( ( 3, 2, 2, 3 ),
 ( 0.000000000000000000, 0.02777777777777779705, 0.05555555555555559410, 0.08333333333333339810 ),
 .UNSPECIFIED. ) 
 CURVE ( )  GEOMETRIC_REPRESENTATION_ITEM ( )  RATIONAL_B_SPLINE_CURVE ( ( 1.000000000000000000, 0.8660254037844387076, 1.000000000000000000, 0.8660254037844387076, 1.000000000000000000, 0.8660254037844383745, 1.000000000000000222 ) ) 
 REPRESENTATION_ITEM ( '' )  );
#9029=CARTESIAN_POINT ( 'NONE',  ( 1.500000000000002887, -12.38667738857996348, -0.03299150346530656946 ) ) ;
#9031=CYLINDRICAL_SURFACE ( 'NONE', #9306, 1.500000000000000222 ) ;
#9061=ORIENTED_EDGE ( 'NONE', *, *, #5898, .T. ) ;
#9062=CARTESIAN_POINT ( 'NONE',  ( -1.229367062500000163, -12.29022459553277002, -1.010416667349463449 ) ) ;
#9071=CARTESIAN_POINT ( 'NONE',  ( 0.7500000000000003331, -11.70096189432334732, -0.9791666680322602678 ) ) ;
#9074=CARTESIAN_POINT ( 'NONE',  ( 0.6146835312500001924, -11.93533689329915326, -1.260416667349463227 ) ) ;
#9083=ADVANCED_FACE ( 'NONE', ( #5292 ), #3698, .F. ) ;
#9088=CARTESIAN_POINT ( 'NONE',  ( 0.6146835312499993043, -14.06466310670085562, -2.302083334016129967 ) ) ;
#9099=ORIENTED_EDGE ( 'NONE', *, *, #885, .T. ) ;
#9101=CARTESIAN_POINT ( 'NONE',  ( -0.6146835312499998594, -11.93533689329915326, -2.677083334016129967 ) ) ;
#9113=CARTESIAN_POINT ( 'NONE',  ( -1.229367062500000385, -13.70977540446723886, -0.9270833340161298564 ) ) ;
#9114=ORIENTED_EDGE ( 'NONE', *, *, #7353, .F. ) ;
#9115=CARTESIAN_POINT ( 'NONE',  ( -1.499999999999998224, -13.86602540378444637, -2.708333333333333037 ) ) ;
#9120=CARTESIAN_POINT ( 'NONE',  ( 0.6146835312499993043, -14.06466310670085562, -0.9270833340161300784 ) ) ;
#9132=CARTESIAN_POINT ( 'NONE',  ( 1.229367062500000163, -13.00000000000000533, -2.718750000682796486 ) ) ;
#9157=CIRCLE ( 'NONE', #7638, 4.000000000000000000 ) ;
#9168=CARTESIAN_POINT ( 'NONE',  ( -2.607672531582950546E-16, -14.41955080893447416, -1.843750000682796708 ) ) ;
#9175=CARTESIAN_POINT ( 'NONE',  ( 1.500000000000000222, -13.00000000000000533, -2.062500001365593416 ) ) ;
#9176=CARTESIAN_POINT ( 'NONE',  ( -2.607672531582950546E-16, -14.41955080893447416, -0.9687500006827967081 ) ) ;
#9182=CARTESIAN_POINT ( 'NONE',  ( 1.060575238724907038E-16, -11.26794919243112680, 0.06249999863440622305 ) ) ;
#9191=CARTESIAN_POINT ( 'NONE',  ( 1.229367062500000163, -13.00000000000000533, -0.7187500006827964860 ) ) ;
#9202=CARTESIAN_POINT ( 'NONE',  ( -1.229367062500000163, -13.00000000000000533, -2.093750000682796930 ) ) ;
#9214=CARTESIAN_POINT ( 'NONE',  ( 1.229367062499999719, -13.70977540446724063, -1.760416667349463227 ) ) ;
#9225=CARTESIAN_POINT ( 'NONE',  ( -1.229367062500000163, -12.29022459553277002, -0.1354166673494631989 ) ) ;
#9241=CARTESIAN_POINT ( 'NONE',  ( 8.692241771943169307E-17, -11.58044919106553294, -2.093750000682796486 ) ) ;
#9244=CARTESIAN_POINT ( 'NONE',  ( 1.229367062500000163, -13.70977540446723886, -0.7604166673494633377 ) ) ;
#9251=ORIENTED_EDGE ( 'NONE', *, *, #6420, .T. ) ;
#9255=CARTESIAN_POINT ( 'NONE',  ( 1.229367062500000385, -12.29022459553277002, -0.3020833340161301339 ) ) ;
#9258=CARTESIAN_POINT ( 'NONE',  ( 1.499999999999996669, -13.86602540378444814, -0.5416666666666670737 ) ) ;
#9274=DIRECTION ( 'NONE',  ( -0.000000000000000000, 1.000000000000000000, 0.000000000000000000 ) ) ;
#9283=CARTESIAN_POINT ( 'NONE',  ( -1.500000000000002220, -12.13397459621556962, -2.791666666666666519 ) ) ;
#9285=CARTESIAN_POINT ( 'NONE',  ( 1.500000000000000222, -12.13397459621556784, -2.020833334698926897 ) ) ;
#9289=CARTESIAN_POINT ( 'NONE',  ( -2.607672531582950546E-16, -14.41955080893447416, -0.8437500006827965970 ) ) ;
#9292=CARTESIAN_POINT ( 'NONE',  ( -0.6146835312499998594, -11.93533689329915326, -1.052083334016129967 ) ) ;
#9304=CARTESIAN_POINT ( 'NONE',  ( 0.6146835312500001924, -11.93533689329915326, -0.7604166673494633377 ) ) ;
#9306=AXIS2_PLACEMENT_3D ( 'NONE', #3940, #7167, #9731 ) ;
#9309=CARTESIAN_POINT ( 'NONE',  ( 1.364683531250000303, -13.00000000000000533, -2.640625001024195395 ) ) ;
#9327=VECTOR ( 'NONE', #5865, 1000.000000000000227 ) ;
#9333=DIRECTION ( 'NONE',  ( 0.000000000000000000, 0.000000000000000000, 1.000000000000000000 ) ) ;
#9336=CARTESIAN_POINT ( 'NONE',  ( -0.7500000000000007772, -14.29903810567666156, -2.229166668032259935 ) ) ;
#9341=CARTESIAN_POINT ( 'NONE',  ( -1.500000000000000222, -13.00000000000000533, -0.2500000000000002220 ) ) ;
#9345=DIRECTION ( 'NONE',  ( 0.000000000000000000, 0.000000000000000000, 1.000000000000000000 ) ) ;
#9347=CARTESIAN_POINT ( 'NONE',  ( -0.6146835312499998594, -11.93533689329915326, -2.177083334016129967 ) ) ;
#9349=CARTESIAN_POINT ( 'NONE',  ( -2.607672531582950546E-16, -14.41955080893447416, -0.8437500006827965970 ) ) ;
#9361=( BOUNDED_CURVE ( )  B_SPLINE_CURVE ( 2, ( #5681, #2127, #2177, #5455, #3129, #7904, #1487 ),
 .UNSPECIFIED., .F., .T. ) 
 B_SPLINE_CURVE_WITH_KNOTS ( ( 3, 2, 2, 3 ),
 ( 0.1666666666666666574, 0.1944444444444444198, 0.2222222222222221544, 0.2499999999999999167 ),
 .UNSPECIFIED. ) 
 CURVE ( )  GEOMETRIC_REPRESENTATION_ITEM ( )  RATIONAL_B_SPLINE_CURVE ( ( 1.000000000000000000, 0.8660254037844387076, 1.000000000000000000, 0.8660254037844387076, 1.000000000000000000, 0.8660254037844391517, 0.9999999999999995559 ) ) 
 REPRESENTATION_ITEM ( '' )  );
#9362=CARTESIAN_POINT ( 'NONE',  ( -1.500000000000000666, -13.86602540378444459, -2.708333333333333481 ) ) ;
#9374=CARTESIAN_POINT ( 'NONE',  ( 1.060575238724907038E-16, -11.26794919243112680, -1.375000000000000222 ) ) ;
#9387=CARTESIAN_POINT ( 'NONE',  ( -0.7499999999999997780, -11.70096189432334555, -0.3958333346989269530 ) ) ;
#9397=CARTESIAN_POINT ( 'NONE',  ( 8.692241771943169307E-17, -11.58044919106553294, -2.718750000682796042 ) ) ;
#9401=CARTESIAN_POINT ( 'NONE',  ( 1.229367062500000163, -13.70977540446723886, -0.2604166673494633377 ) ) ;
#9405=CARTESIAN_POINT ( 'NONE',  ( -3.181725716174720991E-16, -14.73205080756888563, -2.187500001365593416 ) ) ;
#9418=CARTESIAN_POINT ( 'NONE',  ( -2.607672531582950546E-16, -14.41955080893447416, -0.4687500006827967081 ) ) ;
#9445=CARTESIAN_POINT ( 'NONE',  ( 1.500000000000000222, -13.00000000000000533, -1.062500001365593416 ) ) ;
#9454=CARTESIAN_POINT ( 'NONE',  ( 1.229367062500000163, -13.00000000000000533, -0.2187500006827964583 ) ) ;
#9464=CARTESIAN_POINT ( 'NONE',  ( 1.499999999999996669, -13.86602540378444814, -0.1041666680322604899 ) ) ;
#9467=CARTESIAN_POINT ( 'NONE',  ( -0.7499999999999997780, -11.70096189432334555, -2.833333333333333481 ) ) ;
#9473=ORIENTED_EDGE ( 'NONE', *, *, #343, .T. ) ;
#9496=CARTESIAN_POINT ( 'NONE',  ( -0.7499999999999997780, -11.70096189432334555, -2.395833334698926897 ) ) ;
#9500=CYLINDRICAL_SURFACE ( 'NONE', #8893, 4.000000000000000000 ) ;
#9509=CARTESIAN_POINT ( 'NONE',  ( -1.229367062500000385, -13.70977540446723886, 0.07291666598387017140 ) ) ;
#9515=CARTESIAN_POINT ( 'NONE',  ( 0.7499999999999991118, -14.29903810567666333, -2.145833334698926897 ) ) ;
#9521=VERTEX_POINT ( 'NONE', #6191 ) ;
#9526=CARTESIAN_POINT ( 'NONE',  ( -1.500000000000000222, -13.00000000000000533, -1.750000000000000000 ) ) ;
#9530=CYLINDRICAL_SURFACE ( 'NONE', #1366, 1.500000000000000222 ) ;
#9534=LINE ( 'NONE', #8836, #6738 ) ;
#9548=CARTESIAN_POINT ( 'NONE',  ( -0.7500000000000007772, -14.29903810567666156, -1.729166668032260157 ) ) ;
#9557=CARTESIAN_POINT ( 'NONE',  ( 1.500000000000000222, -13.00000000000000533, -2.000000000000000000 ) ) ;
#9562=CARTESIAN_POINT ( 'NONE',  ( -0.6146835312499998594, -11.93533689329915326, -1.677083334016129967 ) ) ;
#9572=CARTESIAN_POINT ( 'NONE',  ( 0.7499999999999991118, -14.29903810567666333, -1.583333333333333481 ) ) ;
#9575=FILL_AREA_STYLE_COLOUR ( '', #1181 ) ;
#9578=CARTESIAN_POINT ( 'NONE',  ( 1.060575238724907038E-16, -11.26794919243112680, -2.374999999999999556 ) ) ;
#9579=PRODUCT_DEFINITION_FORMATION_WITH_SPECIFIED_SOURCE ( 'ANY', '', #7746, .NOT_KNOWN. ) ;
#9588=VERTEX_POINT ( 'NONE', #2173 ) ;
#9594=VERTEX_POINT ( 'NONE', #531 ) ;
#9602=CARTESIAN_POINT ( 'NONE',  ( 1.500000000000000222, -13.00000000000000533, -1.562500001365593416 ) ) ;
#9608=FACE_OUTER_BOUND ( 'NONE', #10172, .T. ) ;
#9617=VECTOR ( 'NONE', #9345, 1000.000000000000000 ) ;
#9628=EDGE_CURVE ( 'NONE', #1061, #1639, #1493, .T. ) ;
#9632=CARTESIAN_POINT ( 'NONE',  ( -1.500000000000000222, -13.00000000000000533, -2.250000000000000444 ) ) ;
#9635=VERTEX_POINT ( 'NONE', #143 ) ;
#9641=ORIENTED_EDGE ( 'NONE', *, *, #7353, .T. ) ;
#9655=CARTESIAN_POINT ( 'NONE',  ( -3.181725716174720498E-16, -14.73205080756888385, -1.187500001365593638 ) ) ;
#9663=CARTESIAN_POINT ( 'NONE',  ( 0.000000000000000000, -13.00000000000000533, -3.000000000000000000 ) ) ;
#9669=CARTESIAN_POINT ( 'NONE',  ( 0.6146835312499993043, -14.06466310670085562, -0.9270833340161300784 ) ) ;
#9690=CARTESIAN_POINT ( 'NONE',  ( -0.7500000000000007772, -14.29903810567666156, -1.166666666666666741 ) ) ;
#9693=EDGE_CURVE ( 'NONE', #9020, #10421, #6154, .T. ) ;
#9700=ORIENTED_EDGE ( 'NONE', *, *, #828, .F. ) ;
#9705=CARTESIAN_POINT ( 'NONE',  ( -1.500000000000000222, -13.00000000000000533, -2.250000000000000444 ) ) ;
#9711=ORIENTED_EDGE ( 'NONE', *, *, #2678, .F. ) ;
#9712=CARTESIAN_POINT ( 'NONE',  ( -1.500000000000000000, -12.13397459621556607, -0.8541666680322602678 ) ) ;
#9722=CARTESIAN_POINT ( 'NONE',  ( -0.6146835312500006365, -14.06466310670085562, -1.010416667349463227 ) ) ;
#9725=AXIS2_PLACEMENT_3D ( 'NONE', #5048, #6731, #8928 ) ;
#9728=CARTESIAN_POINT ( 'NONE',  ( 1.229367062500000163, -13.00000000000000533, 0.1562499993172034307 ) ) ;
#9731=DIRECTION ( 'NONE',  ( 1.000000000000000000, 0.000000000000000000, 0.000000000000000000 ) ) ;
#9732=SHAPE_REPRESENTATION ( 'position sensor magnet', ( #2101 ), #581 ) ;
#9738=CARTESIAN_POINT ( 'NONE',  ( 1.500000000000000222, -13.00000000000000533, -2.000000000000000000 ) ) ;
#9749=ADVANCED_FACE ( 'NONE', ( #2582 ), #2174, .T. ) ;
#9763=CARTESIAN_POINT ( 'NONE',  ( 1.500000000000000000, -13.86602540378444459, -0.1041666680322603095 ) ) ;
#9766=LINE ( 'NONE', #7571, #1433 ) ;
#9768=CARTESIAN_POINT ( 'NONE',  ( 4.000000000000000000, -13.00000000000000533, 2.000000000000000000 ) ) ;
#9769=DIRECTION ( 'NONE',  ( 1.000000000000000000, 0.000000000000000000, 0.000000000000000000 ) ) ;
#9775=CARTESIAN_POINT ( 'NONE',  ( -1.229367062500000163, -12.29022459553277002, -0.6354166673494632267 ) ) ;
#9796=ORIENTED_EDGE ( 'NONE', *, *, #2279, .T. ) ;
#9811=CARTESIAN_POINT ( 'NONE',  ( -1.229367062500000163, -12.29022459553277002, -2.510416667349463449 ) ) ;
#9819=CARTESIAN_POINT ( 'NONE',  ( -0.6146835312499998594, -11.93533689329915326, -1.177083334016129967 ) ) ;
#9822=VECTOR ( 'NONE', #2629, 1000.000000000000000 ) ;
#9823=CARTESIAN_POINT ( 'NONE',  ( -0.6146835312500006365, -14.06466310670085562, -0.5104166673494635598 ) ) ;
#9839=AXIS2_PLACEMENT_3D ( 'NONE', #3430, #9910, #6705 ) ;
#9867=CARTESIAN_POINT ( 'NONE',  ( 0.6146835312499993043, -14.06466310670085562, -1.802083334016129745 ) ) ;
#9873=EDGE_LOOP ( 'NONE', ( #1561, #98, #8962 ) ) ;
#9875=CARTESIAN_POINT ( 'NONE',  ( -2.607672531582950546E-16, -14.41955080893447416, -2.468750000682796930 ) ) ;
#9877=ORIENTED_EDGE ( 'NONE', *, *, #8700, .F. ) ;
#9879=EDGE_CURVE ( 'NONE', #252, #9588, #741, .T. ) ;
#9880=EDGE_CURVE ( 'NONE', #9594, #5863, #4738, .T. ) ;
#9889=CARTESIAN_POINT ( 'NONE',  ( -1.229367062500000385, -13.70977540446723886, -0.9270833340161298564 ) ) ;
#9897=CARTESIAN_POINT ( 'NONE',  ( -1.500000000000000222, -13.00000000000000533, -2.750000000000000000 ) ) ;
#9898=ORIENTED_EDGE ( 'NONE', *, *, #8502, .T. ) ;
#9900=LINE ( 'NONE', #4208, #9822 ) ;
#9909=DIRECTION ( 'NONE',  ( 0.000000000000000000, 0.000000000000000000, 1.000000000000000000 ) ) ;
#9910=DIRECTION ( 'NONE',  ( 0.000000000000000000, 0.000000000000000000, 1.000000000000000000 ) ) ;
#9917=CARTESIAN_POINT ( 'NONE',  ( -0.6146835312499998594, -11.93533689329915326, -1.052083334016129967 ) ) ;
#9928=CARTESIAN_POINT ( 'NONE',  ( 8.692241771943170539E-17, -11.58044919106553650, -1.718750000682796708 ) ) ;
#9945=CARTESIAN_POINT ( 'NONE',  ( 1.229367062500000163, -13.70977540446723886, -2.260416667349463449 ) ) ;
#9969=CARTESIAN_POINT ( 'NONE',  ( -1.229367062500000163, -13.00000000000000533, -0.4687500006827967081 ) ) ;
#9973=DIRECTION ( 'NONE',  ( 0.000000000000000000, 0.000000000000000000, 1.000000000000000000 ) ) ;
#9976=CARTESIAN_POINT ( 'NONE',  ( -0.6146835312500006365, -14.06466310670085562, -0.5104166673494635598 ) ) ;
#9987=CARTESIAN_POINT ( 'NONE',  ( -0.7499999999999997780, -11.70096189432334555, -1.895833334698926897 ) ) ;
#9992=CARTESIAN_POINT ( 'NONE',  ( -2.607672531582950546E-16, -14.41955080893447416, -1.343750000682796708 ) ) ;
#9997=ADVANCED_FACE ( 'NONE', ( #7910 ), #8702, .T. ) ;
#10007=CARTESIAN_POINT ( 'NONE',  ( -0.6146835312499998594, -11.93533689329915326, -2.177083334016129967 ) ) ;
#10015=APPLICATION_CONTEXT ( 'automotive_design' ) ;
#10024=CARTESIAN_POINT ( 'NONE',  ( 1.229367062499999719, -13.70977540446724063, -0.2604166673494632822 ) ) ;
#10031=DIRECTION ( 'NONE',  ( 0.000000000000000000, 0.000000000000000000, 1.000000000000000000 ) ) ;
#10035=CARTESIAN_POINT ( 'NONE',  ( 8.692241771943170539E-17, -11.58044919106553650, -2.218750000682796486 ) ) ;
#10039=ADVANCED_FACE ( 'NONE', ( #3403, #8968 ), #8180, .F. ) ;
#10045=FACE_OUTER_BOUND ( 'NONE', #7549, .T. ) ;
#10047=CARTESIAN_POINT ( 'NONE',  ( -1.229367062500000385, -13.70977540446723886, -2.427083334016129967 ) ) ;
#10049=CARTESIAN_POINT ( 'NONE',  ( 8.692241771943170539E-17, -11.58044919106553650, -0.09375000068279679133 ) ) ;
#10057=AXIS2_PLACEMENT_3D ( 'NONE', #2241, #10363, #3988 ) ;
#10060=CARTESIAN_POINT ( 'NONE',  ( -0.6146835312499998594, -11.93533689329915326, -1.677083334016129967 ) ) ;
#10071=ORIENTED_EDGE ( 'NONE', *, *, #9879, .F. ) ;
#10076=COLOUR_RGB ( '', 0.09019608, 0.27058824, 0.51372549) ;
#10089=CARTESIAN_POINT ( 'NONE',  ( -1.499999999999999778, -12.13397459621556784, 0.1458333319677399265 ) ) ;
#10090=CARTESIAN_POINT ( 'NONE',  ( 1.500000000000000222, -13.00000000000000533, -3.000000000000000000 ) ) ;
#10096=CARTESIAN_POINT ( 'NONE',  ( 8.692241771943169307E-17, -11.58044919106553294, -2.593750000682796486 ) ) ;
#10099=CARTESIAN_POINT ( 'NONE',  ( -0.6146835312500006365, -14.06466310670085562, -1.885416667349463227 ) ) ;
#10110=( BOUNDED_SURFACE ( )  B_SPLINE_SURFACE ( 1, 2, ( 
 ( #9132, #5983, #8397, #10096, #6728, #5200, #2619, #10047, #5257, #6686, #9088, #334, #2770, #3612, #1076, #9241, #1229, #1822, #4298, #2030, #3665, #1874, #5882, #7649, #4249, #439, #2823, #7543, #8294, #1020, #289, #3512, #7494, #9992, #2667, #5149, #5936, #4351, #1128, #6036, #7591, #1980, #3562, #9889, #1176, #9289, #8498, #4454, #6095, #1438, #10248, #2183, #3819, #2081, #3083, #4508, #6893, #2928, #6996, #5307, #9454, #5460, #8597, #2239, #8699, #1282, #639, #9509, #1328, #2981, #700, #4558, #7048 ),
 ( #6200, #4662, #7806, #9397, #5407, #7854, #10202, #3870, #8548, #588, #10146, #7102, #8650, #7753, #6147, #4610, #9347, #7908, #3029, #2870, #10359, #487, #1386, #6303, #3714, #540, #3767, #10300, #9562, #6945, #6250, #2134, #5356, #2289, #5515, #4714, #8753, #1492, #7963, #2399, #8124, #910, #8864, #3134, #9722, #860, #9669, #3189, #6410, #66, #2453, #4136, #806, #9775, #7156, #4089, #9823, #8020, #10413, #4879, #7323, #4937, #5619, #3292, #5771, #6362, #1605, #6571, #8232, #4828, #10470, #8964, #8809 ) ),
 .UNSPECIFIED., .F., .F., .T. ) 
 B_SPLINE_SURFACE_WITH_KNOTS ( ( 2, 2 ),
 ( 3, 2, 2, 2, 2, 2, 2, 2, 2, 2, 2, 2, 2, 2, 2, 2, 2, 2, 2, 2, 2, 2, 2, 2, 2, 2, 2, 2, 2, 2, 2, 2, 2, 2, 2, 2, 3 ),
 ( 0.000000000000000000, 1.000000000000000000 ),
 ( 0.000000000000000000, 0.02777777777777777624, 0.05555555555555555247, 0.08333333333333332871, 0.1111111111111111049, 0.1388888888888888951, 0.1666666666666666574, 0.1944444444444444475, 0.2222222222222222099, 0.2500000000000000000, 0.2777777777777777901, 0.3055555555555555802, 0.3333333333333333148, 0.3611111111111111049, 0.3888888888888888951, 0.4166666666666666852, 0.4444444444444444198, 0.4722222222222222099, 0.5000000000000000000, 0.5277777777777777901, 0.5555555555555555802, 0.5833333333333333703, 0.6111111111111111605, 0.6388888888888888395, 0.6666666666666666297, 0.6944444444444444198, 0.7222222222222222099, 0.7500000000000000000, 0.7777777777777777901, 0.8055555555555555802, 0.8333333333333333703, 0.8611111111111111605, 0.8888888888888888395, 0.9166666666666666297, 0.9444444444444444198, 0.9722222222222222099, 1.000000000000000000 ),
 .UNSPECIFIED. ) 
 GEOMETRIC_REPRESENTATION_ITEM ( )  RATIONAL_B_SPLINE_SURFACE ( (
 ( 1.000000000000000000, 0.8660254037844387076, 1.000000000000000000, 0.8660254037844387076, 1.000000000000000000, 0.8660254037844387076, 1.000000000000000000, 0.8660254037844387076, 1.000000000000000000, 0.8660254037844387076, 1.000000000000000000, 0.8660254037844387076, 1.000000000000000000, 0.8660254037844387076, 1.000000000000000000, 0.8660254037844387076, 1.000000000000000000, 0.8660254037844387076, 1.000000000000000000, 0.8660254037844387076, 1.000000000000000000, 0.8660254037844387076, 1.000000000000000000, 0.8660254037844387076, 1.000000000000000000, 0.8660254037844387076, 1.000000000000000000, 0.8660254037844387076, 1.000000000000000000, 0.8660254037844387076, 1.000000000000000000, 0.8660254037844387076, 1.000000000000000000, 0.8660254037844387076, 1.000000000000000000, 0.8660254037844387076, 1.000000000000000000, 0.8660254037844387076, 1.000000000000000000, 0.8660254037844387076, 1.000000000000000000, 0.8660254037844387076, 1.000000000000000000, 0.8660254037844387076, 1.000000000000000000, 0.8660254037844387076, 1.000000000000000000, 0.8660254037844387076, 1.000000000000000000, 0.8660254037844387076, 1.000000000000000000, 0.8660254037844387076, 1.000000000000000000, 0.8660254037844387076, 1.000000000000000000, 0.8660254037844387076, 1.000000000000000000, 0.8660254037844387076, 1.000000000000000000, 0.8660254037844387076, 1.000000000000000000, 0.8660254037844387076, 1.000000000000000000, 0.8660254037844387076, 1.000000000000000000, 0.8660254037844387076, 1.000000000000000000, 0.8660254037844387076, 1.000000000000000000, 0.8660254037844387076, 1.000000000000000000, 0.8660254037844387076, 1.000000000000000000),
 ( 1.000000000000000000, 0.8660254037844387076, 1.000000000000000000, 0.8660254037844387076, 1.000000000000000000, 0.8660254037844387076, 1.000000000000000000, 0.8660254037844387076, 1.000000000000000000, 0.8660254037844387076, 1.000000000000000000, 0.8660254037844387076, 1.000000000000000000, 0.8660254037844387076, 1.000000000000000000, 0.8660254037844387076, 1.000000000000000000, 0.8660254037844387076, 1.000000000000000000, 0.8660254037844387076, 1.000000000000000000, 0.8660254037844387076, 1.000000000000000000, 0.8660254037844387076, 1.000000000000000000, 0.8660254037844387076, 1.000000000000000000, 0.8660254037844387076, 1.000000000000000000, 0.8660254037844387076, 1.000000000000000000, 0.8660254037844387076, 1.000000000000000000, 0.8660254037844387076, 1.000000000000000000, 0.8660254037844387076, 1.000000000000000000, 0.8660254037844387076, 1.000000000000000000, 0.8660254037844387076, 1.000000000000000000, 0.8660254037844387076, 1.000000000000000000, 0.8660254037844387076, 1.000000000000000000, 0.8660254037844387076, 1.000000000000000000, 0.8660254037844387076, 1.000000000000000000, 0.8660254037844387076, 1.000000000000000000, 0.8660254037844387076, 1.000000000000000000, 0.8660254037844387076, 1.000000000000000000, 0.8660254037844387076, 1.000000000000000000, 0.8660254037844387076, 1.000000000000000000, 0.8660254037844387076, 1.000000000000000000, 0.8660254037844387076, 1.000000000000000000, 0.8660254037844387076, 1.000000000000000000, 0.8660254037844387076, 1.000000000000000000, 0.8660254037844387076, 1.000000000000000000, 0.8660254037844387076, 1.000000000000000000, 0.8660254037844387076, 1.000000000000000000) ) ) 
 REPRESENTATION_ITEM ( '' )  SURFACE ( )  );
#10111=CARTESIAN_POINT ( 'NONE',  ( 1.229367062499999719, -13.70977540446724063, 0.1145833326505365929 ) ) ;
#10137=CARTESIAN_POINT ( 'NONE',  ( 1.500000000000000444, -12.13397459621556607, -2.520833334698926897 ) ) ;
#10146=CARTESIAN_POINT ( 'NONE',  ( 0.6146835312499993043, -14.06466310670085562, -2.427083334016129967 ) ) ;
#10158=( NAMED_UNIT ( * ) SI_UNIT ( $, .STERADIAN. ) SOLID_ANGLE_UNIT ( ) );
#10161=CARTESIAN_POINT ( 'NONE',  ( -0.6146835312499998594, -11.93533689329915326, -1.177083334016129967 ) ) ;
#10172=EDGE_LOOP ( 'NONE', ( #8656, #9898, #7346, #3018 ) ) ;
#10189=FACE_OUTER_BOUND ( 'NONE', #8428, .T. ) ;
#10193=CARTESIAN_POINT ( 'NONE',  ( -1.500000000000000222, -13.00000000000000533, 0.1874999986344063341 ) ) ;
#10202=CARTESIAN_POINT ( 'NONE',  ( -1.229367062500000163, -13.00000000000000533, -2.593750000682796486 ) ) ;
#10204=CARTESIAN_POINT ( 'NONE',  ( 8.692241771943170539E-17, -11.58044919106553650, -0.5937500006827968191 ) ) ;
#10215=CARTESIAN_POINT ( 'NONE',  ( -1.229367062500000163, -13.00000000000000533, -0.5937500006827968191 ) ) ;
#10221=ORIENTED_EDGE ( 'NONE', *, *, #5695, .F. ) ;
#10238=CARTESIAN_POINT ( 'NONE',  ( 0.7500000000000003331, -11.70096189432334732, -2.479166668032260379 ) ) ;
#10241=CARTESIAN_POINT ( 'NONE',  ( 1.500000000000000222, -12.13397459621556784, -2.958333333333333037 ) ) ;
#10248=CARTESIAN_POINT ( 'NONE',  ( 0.6146835312500001924, -11.93533689329915326, -0.6354166673494632267 ) ) ;
#10251=CARTESIAN_POINT ( 'NONE',  ( -0.6146835312499998594, -11.93533689329915326, -1.552083334016129967 ) ) ;
#10260=DIRECTION ( 'NONE',  ( 0.000000000000000000, 0.000000000000000000, 1.000000000000000000 ) ) ;
#10266=CARTESIAN_POINT ( 'NONE',  ( -1.229367062500000163, -12.29022459553277002, -0.1354166673494631989 ) ) ;
#10270=VERTEX_POINT ( 'NONE', #5348 ) ;
#10278=CARTESIAN_POINT ( 'NONE',  ( 1.500000000000000222, -13.00000000000000533, -1.562500001365593416 ) ) ;
#10285=CARTESIAN_POINT ( 'NONE',  ( 4.000000000000000000, -13.00000000000000533, 0.000000000000000000 ) ) ;
#10289=CARTESIAN_POINT ( 'NONE',  ( -3.181725716174720498E-16, -14.73205080756888385, -2.187500001365593416 ) ) ;
#10300=CARTESIAN_POINT ( 'NONE',  ( 8.692241771943169307E-17, -11.58044919106553294, -1.718750000682796708 ) ) ;
#10308=CARTESIAN_POINT ( 'NONE',  ( 1.500000000000000222, -13.00000000000000533, -1.500000000000000000 ) ) ;
#10313=CARTESIAN_POINT ( 'NONE',  ( -1.500000000000000666, -13.86602540378444459, -2.208333333333333481 ) ) ;
#10318=CARTESIAN_POINT ( 'NONE',  ( -0.7499999999999997780, -11.70096189432334555, -2.395833334698926897 ) ) ;
#10325=EDGE_CURVE ( 'NONE', #8892, #2098, #2581, .T. ) ;
#10332=( NAMED_UNIT ( * ) SI_UNIT ( $, .STERADIAN. ) SOLID_ANGLE_UNIT ( ) );
#10338=ORIENTED_EDGE ( 'NONE', *, *, #885, .F. ) ;
#10345=CARTESIAN_POINT ( 'NONE',  ( -1.500000000000000222, -13.00000000000000533, -1.812500001365593416 ) ) ;
#10353=CARTESIAN_POINT ( 'NONE',  ( -1.500000000000003331, -13.86602540378444104, -2.208333333333333481 ) ) ;
#10359=CARTESIAN_POINT ( 'NONE',  ( -0.6146835312500006365, -14.06466310670085562, -2.010416667349463005 ) ) ;
#10363=DIRECTION ( 'NONE',  ( 0.000000000000000000, 0.000000000000000000, 1.000000000000000000 ) ) ;
#10376=CARTESIAN_POINT ( 'NONE',  ( -0.7499999999999997780, -11.70096189432334555, -1.833333333333333481 ) ) ;
#10402=CARTESIAN_POINT ( 'NONE',  ( 1.060575238724907038E-16, -11.26794919243112680, -0.9375000013655937492 ) ) ;
#10407=CARTESIAN_POINT ( 'NONE',  ( 0.000000000000000000, -13.00000000000000533, 2.000000000000000000 ) ) ;
#10413=CARTESIAN_POINT ( 'NONE',  ( 0.6146835312499993043, -14.06466310670085562, -0.4270833340161298564 ) ) ;
#10421=VERTEX_POINT ( 'NONE', #9445 ) ;
#10426=CARTESIAN_POINT ( 'NONE',  ( 1.500000000000000222, -13.00000000000000533, -0.06250000136559345776 ) ) ;
#10430=CARTESIAN_POINT ( 'NONE',  ( 0.7500000000000003331, -11.70096189432334732, -2.416666666666666963 ) ) ;
#10434=ORIENTED_EDGE ( 'NONE', *, *, #5006, .T. ) ;
#10438=EDGE_CURVE ( 'NONE', #9594, #10270, #2175, .T. ) ;
#10440=FACE_OUTER_BOUND ( 'NONE', #3273, .T. ) ;
#10451=CARTESIAN_POINT ( 'NONE',  ( 0.7500000000000003331, -11.70096189432334732, -1.916666666666666741 ) ) ;
#10457=CARTESIAN_POINT ( 'NONE',  ( 1.229367062500000163, -13.00000000000000533, -2.718750000682796486 ) ) ;
#10458=CARTESIAN_POINT ( 'NONE',  ( 1.229367062500000385, -12.29022459553277002, -2.302083334016129967 ) ) ;
#10460=( BOUNDED_CURVE ( )  B_SPLINE_CURVE ( 2, ( #3250, #9029, #4836 ),
 .UNSPECIFIED., .F., .T. ) 
 B_SPLINE_CURVE_WITH_KNOTS ( ( 3, 3 ),
 ( 0.8333333333333332593, 0.8538060088535064374 ),
 .UNSPECIFIED. ) 
 CURVE ( )  GEOMETRIC_REPRESENTATION_ITEM ( )  RATIONAL_B_SPLINE_CURVE ( ( 1.000000000000000444, 0.9012585362943735801, 0.9480652127606681301 ) ) 
 REPRESENTATION_ITEM ( '' )  );
#10465=FACE_OUTER_BOUND ( 'NONE', #2295, .T. ) ;
#10470=CARTESIAN_POINT ( 'NONE',  ( 0.6146835312499993043, -14.06466310670085562, 0.07291666598386974119 ) ) ;
#10477=DIRECTION ( 'NONE',  ( 1.000000000000000000, 0.000000000000000000, 0.000000000000000000 ) ) ;
#10478=CYLINDRICAL_SURFACE ( 'NONE', #5679, 4.000000000000000000 ) ;
#10481=CARTESIAN_POINT ( 'NONE',  ( 1.500000000000000222, -13.00000000000000533, -3.000000000000000000 ) ) ;
#10488=CARTESIAN_POINT ( 'NONE',  ( -0.7499999999999997780, -11.70096189432334555, -0.3333333333333334814 ) ) ;
#10498=CARTESIAN_POINT ( 'NONE',  ( -1.500000000000000666, -13.86602540378444459, -0.7708333346989267865 ) ) ;
ENDSEC;
END-ISO-10303-21;
